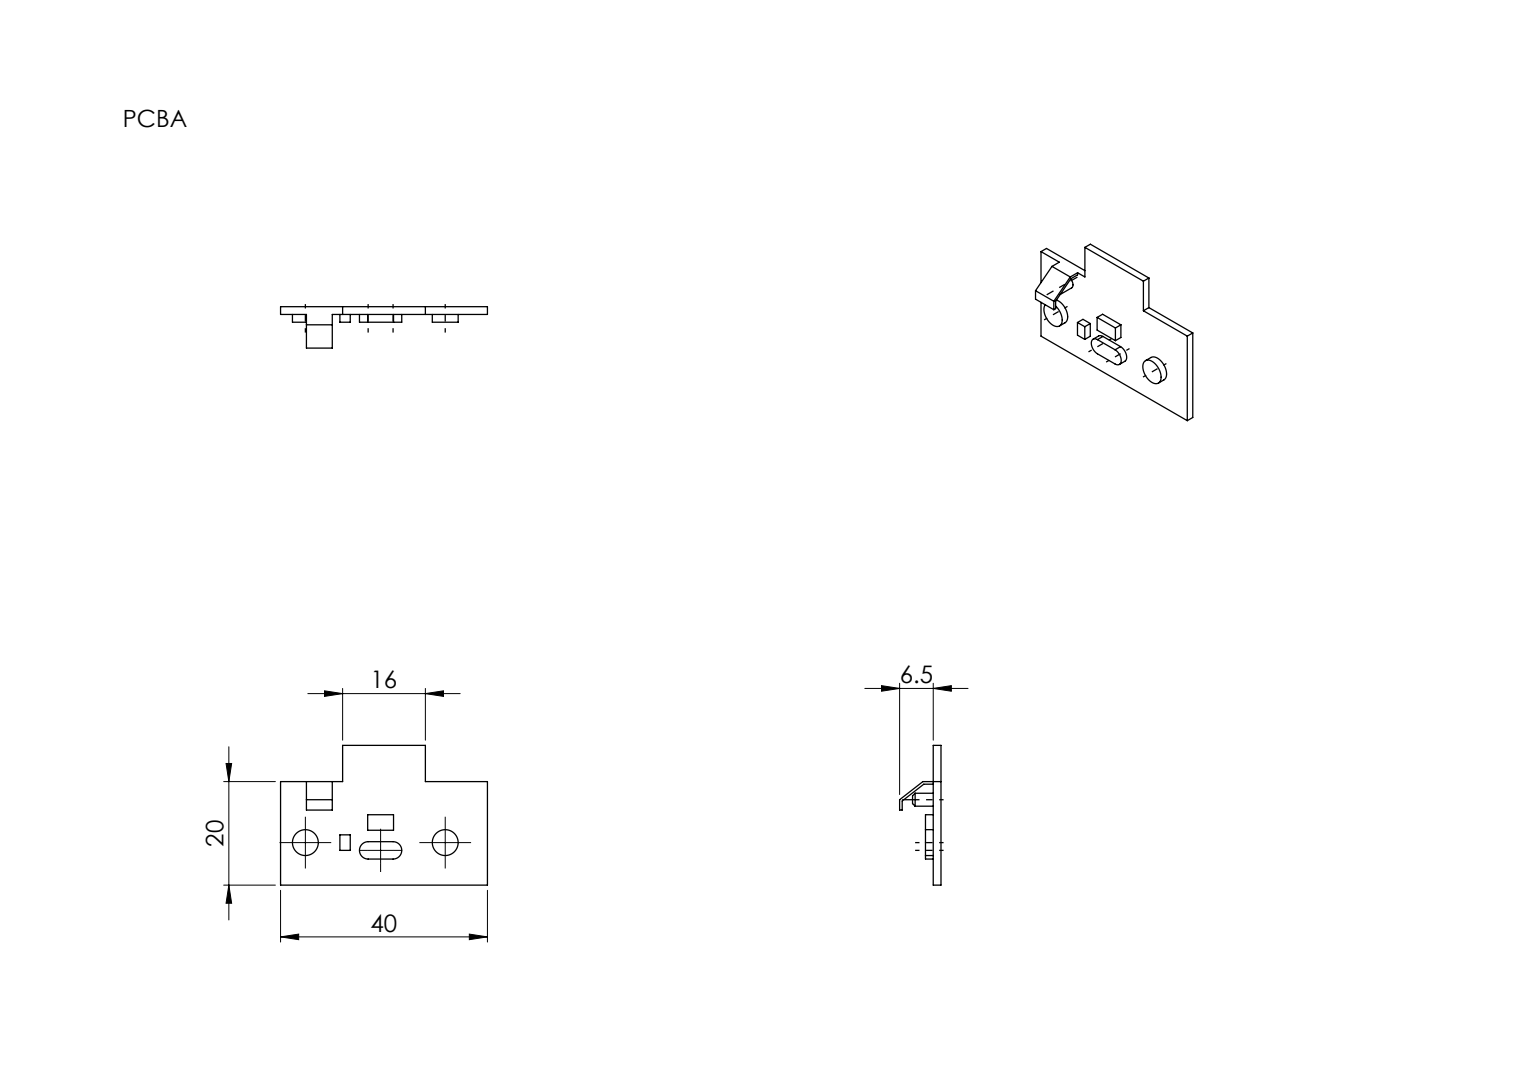
ISO-10303-21;
HEADER;
FILE_DESCRIPTION (('STEP AP214'),
    '1' );
FILE_NAME ('pcba.step',
    '2026-10-08T14:41:38',
    ( '' ),
    ( '' ),
    'SwSTEP 2.0',
    'SolidWorks 2026',
    '' );
FILE_SCHEMA (( 'AUTOMOTIVE_DESIGN' ));
ENDSEC;

DATA;
#13=DIRECTION ( 'NONE',  ( -1.000000000000000000, -2.168404344971008868E-16, 0.000000000000000000 ) ) ;
#56=ADVANCED_FACE ( 'NONE', ( #13399 ), #17297, .T. ) ;
#65=DIRECTION ( 'NONE',  ( 1.000000000000000000, 0.000000000000000000, 0.000000000000000000 ) ) ;
#70=LINE ( 'NONE', #3095, #14117 ) ;
#72=VERTEX_POINT ( 'NONE', #4700 ) ;
#100=EDGE_LOOP ( 'NONE', ( #14836, #13611, #8992, #9930 ) ) ;
#134=DIRECTION ( 'NONE',  ( 0.000000000000000000, -1.000000000000000000, 0.000000000000000000 ) ) ;
#136=AXIS2_PLACEMENT_3D ( 'NONE', #17568, #5609, #6979 ) ;
#169=ADVANCED_FACE ( 'NONE', ( #13798 ), #17134, .T. ) ;
#190=ADVANCED_FACE ( 'NONE', ( #565 ), #6556, .T. ) ;
#192=AXIS2_PLACEMENT_3D ( 'NONE', #9179, #627, #10638 ) ;
#199=DIRECTION ( 'NONE',  ( 0.000000000000000000, 1.000000000000000000, -0.000000000000000000 ) ) ;
#210=CIRCLE ( 'NONE', #18070, 1.678500596222258556 ) ;
#241=UNCERTAINTY_MEASURE_WITH_UNIT (LENGTH_MEASURE( 1.000000000000000082E-05 ), #5755, 'distance_accuracy_value', 'NONE');
#281=LINE ( 'NONE', #12431, #10985 ) ;
#287=EDGE_LOOP ( 'NONE', ( #9707, #2750, #19384, #14817 ) ) ;
#301=VERTEX_POINT ( 'NONE', #18229 ) ;
#308=CARTESIAN_POINT ( 'NONE',  ( -3.155775640247338920, -41.39960408384398249, 3.000000000000000000 ) ) ;
#326=VECTOR ( 'NONE', #8831, 1000.000000000000000 ) ;
#330=EDGE_LOOP ( 'NONE', ( #1279, #8353, #4314, #6562 ) ) ;
#363=EDGE_LOOP ( 'NONE', ( #16148, #12127, #5971, #7441 ) ) ;
#376=ORIENTED_EDGE ( 'NONE', *, *, #4655, .F. ) ;
#414=CARTESIAN_POINT ( 'NONE',  ( -15.20357423236093375, -43.78611686177728046, 3.000000000000000000 ) ) ;
#440=ORIENTED_EDGE ( 'NONE', *, *, #14376, .F. ) ;
#446=DIRECTION ( 'NONE',  ( -1.000000000000000000, 0.000000000000000000, -0.000000000000000000 ) ) ;
#452=LINE ( 'NONE', #1930, #15081 ) ;
#456=DIRECTION ( 'NONE',  ( -0.000000000000000000, -0.000000000000000000, -1.000000000000000000 ) ) ;
#471=DIRECTION ( 'NONE',  ( 0.000000000000000000, -1.000000000000000000, 0.000000000000000000 ) ) ;
#492=ORIENTED_EDGE ( 'NONE', *, *, #2758, .T. ) ;
#507=DIRECTION ( 'NONE',  ( 0.000000000000000000, -1.000000000000000000, 0.000000000000000000 ) ) ;
#508=CARTESIAN_POINT ( 'NONE',  ( 20.00000000000000355, -32.00000000000000711, 1.500000000000000000 ) ) ;
#519=CARTESIAN_POINT ( 'NONE',  ( -10.00000000000000000, -17.18313764714974923, -16.36466261444977377 ) ) ;
#558=DIRECTION ( 'NONE',  ( -1.000000000000000000, 0.000000000000000000, -0.000000000000000000 ) ) ;
#565=FACE_OUTER_BOUND ( 'NONE', #15076, .T. ) ;
#567=DIRECTION ( 'NONE',  ( 0.000000000000000000, 1.000000000000000000, 0.000000000000000000 ) ) ;
#573=ORIENTED_EDGE ( 'NONE', *, *, #9984, .T. ) ;
#578=VERTEX_POINT ( 'NONE', #19174 ) ;
#614=ORIENTED_EDGE ( 'NONE', *, *, #3279, .F. ) ;
#627=DIRECTION ( 'NONE',  ( 0.000000000000000000, 0.000000000000000000, 1.000000000000000000 ) ) ;
#747=CARTESIAN_POINT ( 'NONE',  ( 0.000000000000000000, 0.000000000000000000, 3.000000000000000000 ) ) ;
#752=CARTESIAN_POINT ( 'NONE',  ( -1.485306817036799787, -32.50000000000000711, -3.000000000000000000 ) ) ;
#754=DIRECTION ( 'NONE',  ( 1.000000000000000000, 0.000000000000000000, 0.000000000000000000 ) ) ;
#763=VERTEX_POINT ( 'NONE', #6340 ) ;
#793=VERTEX_POINT ( 'NONE', #18588 ) ;
#811=SURFACE_SIDE_STYLE ('',( #2189 ) ) ;
#826=LINE ( 'NONE', #14446, #4346 ) ;
#833=DIRECTION ( 'NONE',  ( -0.000000000000000000, -0.000000000000000000, -1.000000000000000000 ) ) ;
#850=CARTESIAN_POINT ( 'NONE',  ( -12.50000000000000000, -35.50000000000000000, 5.500000000000000000 ) ) ;
#856=VERTEX_POINT ( 'NONE', #12774 ) ;
#873=PLANE ( 'NONE',  #1854 ) ;
#874=PLANE ( 'NONE',  #924 ) ;
#878=CARTESIAN_POINT ( 'NONE',  ( -6.528048594804060301, -45.28611686177728046, 3.000000000000000000 ) ) ;
#893=EDGE_LOOP ( 'NONE', ( #6187, #11365, #9315, #5304 ) ) ;
#924=AXIS2_PLACEMENT_3D ( 'NONE', #9416, #11075, #6488 ) ;
#938=EDGE_LOOP ( 'NONE', ( #12819, #19041, #5593, #2064 ) ) ;
#947=VECTOR ( 'NONE', #14495, 1000.000000000000000 ) ;
#961=LINE ( 'NONE', #13293, #11013 ) ;
#974=FACE_OUTER_BOUND ( 'NONE', #10751, .T. ) ;
#988=EDGE_CURVE ( 'NONE', #18409, #8629, #826, .T. ) ;
#997=CARTESIAN_POINT ( 'NONE',  ( -6.528048594804062965, -42.28611686177728046, 3.000000000000000000 ) ) ;
#1008=DIRECTION ( 'NONE',  ( 0.000000000000000000, 0.000000000000000000, 1.000000000000000000 ) ) ;
#1021=DIRECTION ( 'NONE',  ( -1.000000000000000000, -0.000000000000000000, -0.000000000000000000 ) ) ;
#1027=DIRECTION ( 'NONE',  ( 0.000000000000000000, -0.000000000000000000, 1.000000000000000000 ) ) ;
#1060=ADVANCED_FACE ( 'NONE', ( #19255 ), #2675, .F. ) ;
#1110=EDGE_CURVE ( 'NONE', #18251, #11621, #16207, .T. ) ;
#1111=CARTESIAN_POINT ( 'NONE',  ( 1.844224359752661968, -41.39960408384398249, 3.000000000000000000 ) ) ;
#1239=CARTESIAN_POINT ( 'NONE',  ( -15.00000000000000000, -32.00000000000000711, 1.500000000000000000 ) ) ;
#1246=ORIENTED_EDGE ( 'NONE', *, *, #7374, .T. ) ;
#1269=DIRECTION ( 'NONE',  ( -0.000000000000000000, -0.000000000000000000, -1.000000000000000000 ) ) ;
#1279=ORIENTED_EDGE ( 'NONE', *, *, #12979, .F. ) ;
#1294=VECTOR ( 'NONE', #5042, 1000.000000000000000 ) ;
#1303=CARTESIAN_POINT ( 'NONE',  ( -15.00000000000000000, -32.50000000000000711, -3.000000000000000000 ) ) ;
#1311=DIRECTION ( 'NONE',  ( -1.000000000000000000, -0.000000000000000000, -0.000000000000000000 ) ) ;
#1316=CARTESIAN_POINT ( 'NONE',  ( 20.00000000000000355, -32.00000000000000711, 1.500000000000000000 ) ) ;
#1345=EDGE_LOOP ( 'NONE', ( #11317, #15399, #5466, #15948 ) ) ;
#1361=EDGE_CURVE ( 'NONE', #8629, #9506, #8151, .T. ) ;
#1366=ADVANCED_FACE ( 'NONE', ( #8332 ), #874, .F. ) ;
#1372=VERTEX_POINT ( 'NONE', #16983 ) ;
#1403=CARTESIAN_POINT ( 'NONE',  ( -1.485306817036799787, -32.50000000000001421, 3.328446124929187455 ) ) ;
#1407=ORIENTED_EDGE ( 'NONE', *, *, #2893, .F. ) ;
#1412=CARTESIAN_POINT ( 'NONE',  ( 0.000000000000000000, -32.00000000000000711, 1.500000000000000000 ) ) ;
#1413=ADVANCED_FACE ( 'NONE', ( #974 ), #5772, .F. ) ;
#1420=AXIS2_PLACEMENT_3D ( 'NONE', #8834, #4433, #7561 ) ;
#1430=AXIS2_PLACEMENT_3D ( 'NONE', #414, #15121, #12459 ) ;
#1446=DIRECTION ( 'NONE',  ( 0.000000000000000000, -1.000000000000000000, 0.000000000000000000 ) ) ;
#1482=LINE ( 'NONE', #6087, #16267 ) ;
#1488=ORIENTED_EDGE ( 'NONE', *, *, #13083, .F. ) ;
#1515=FACE_OUTER_BOUND ( 'NONE', #9786, .T. ) ;
#1530=DIRECTION ( 'NONE',  ( -0.000000000000000000, -0.000000000000000000, -1.000000000000000000 ) ) ;
#1538=CARTESIAN_POINT ( 'NONE',  ( -1.485306817036799787, -37.50000000000000000, 7.999999999999996447 ) ) ;
#1545=FACE_OUTER_BOUND ( 'NONE', #11575, .T. ) ;
#1569=EDGE_CURVE ( 'NONE', #18409, #6170, #16064, .T. ) ;
#1585=LINE ( 'NONE', #2849, #326 ) ;
#1612=FACE_OUTER_BOUND ( 'NONE', #16172, .T. ) ;
#1614=DIRECTION ( 'NONE',  ( 0.000000000000000000, -0.000000000000000000, -1.000000000000000000 ) ) ;
#1647=VERTEX_POINT ( 'NONE', #6265 ) ;
#1676=CYLINDRICAL_SURFACE ( 'NONE', #9076, 1.678500596222258556 ) ;
#1707=CYLINDRICAL_SURFACE ( 'NONE', #11087, 2.500000000000000444 ) ;
#1709=CARTESIAN_POINT ( 'NONE',  ( 8.000000000000003553, -25.00000000000000711, 0.000000000000000000 ) ) ;
#1764=ORIENTED_EDGE ( 'NONE', *, *, #10465, .T. ) ;
#1791=AXIS2_PLACEMENT_3D ( 'NONE', #13713, #4815, #7646 ) ;
#1792=DIRECTION ( 'NONE',  ( -0.000000000000000000, -1.000000000000000000, -0.000000000000000000 ) ) ;
#1802=CARTESIAN_POINT ( 'NONE',  ( -7.999999999999996447, 0.000000000000000000, 1.500000000000000000 ) ) ;
#1821=CARTESIAN_POINT ( 'NONE',  ( -10.00000000000000000, -32.00000000000000711, -3.000000000000000000 ) ) ;
#1826=CARTESIAN_POINT ( 'NONE',  ( 9.339266095310328808, -43.78611686177728046, 3.000000000000000000 ) ) ;
#1842=ORIENTED_EDGE ( 'NONE', *, *, #1110, .T. ) ;
#1846=EDGE_LOOP ( 'NONE', ( #6833, #19010 ) ) ;
#1849=CARTESIAN_POINT ( 'NONE',  ( -8.528048594804062077, -45.28611686177728046, 1.500000000000000000 ) ) ;
#1851=ADVANCED_FACE ( 'NONE', ( #15380 ), #1951, .T. ) ;
#1854=AXIS2_PLACEMENT_3D ( 'NONE', #6851, #17256, #7042 ) ;
#1864=ORIENTED_EDGE ( 'NONE', *, *, #15200, .T. ) ;
#1868=DIRECTION ( 'NONE',  ( -1.000000000000000000, 0.000000000000000000, 0.000000000000000000 ) ) ;
#1881=VECTOR ( 'NONE', #2671, 1000.000000000000000 ) ;
#1899=ORIENTED_EDGE ( 'NONE', *, *, #3507, .T. ) ;
#1900=VECTOR ( 'NONE', #1311, 1000.000000000000000 ) ;
#1930=CARTESIAN_POINT ( 'NONE',  ( -15.00000000000000000, 0.000000000000000000, 7.499999999999995559 ) ) ;
#1948=ORIENTED_EDGE ( 'NONE', *, *, #18362, .F. ) ;
#1951=PLANE ( 'NONE',  #9058 ) ;
#1972=ORIENTED_EDGE ( 'NONE', *, *, #16364, .F. ) ;
#1981=CARTESIAN_POINT ( 'NONE',  ( -6.528048594804062965, -42.28611686177728046, 1.500000000000000000 ) ) ;
#2003=EDGE_CURVE ( 'NONE', #6543, #16247, #14565, .T. ) ;
#2024=EDGE_LOOP ( 'NONE', ( #17054, #11269, #614, #1864 ) ) ;
#2052=VERTEX_POINT ( 'NONE', #10135 ) ;
#2064=ORIENTED_EDGE ( 'NONE', *, *, #8373, .F. ) ;
#2076=LINE ( 'NONE', #12065, #18989 ) ;
#2083=CARTESIAN_POINT ( 'NONE',  ( 0.000000000000000000, -32.00000000000000711, 1.500000000000000000 ) ) ;
#2100=AXIS2_PLACEMENT_3D ( 'NONE', #12458, #507, #9517 ) ;
#2118=DIRECTION ( 'NONE',  ( 8.673617379884027583E-16, -1.000000000000000000, 0.000000000000000000 ) ) ;
#2133=ORIENTED_EDGE ( 'NONE', *, *, #10715, .T. ) ;
#2157=EDGE_LOOP ( 'NONE', ( #18218, #13220, #5391, #13980, #3183 ) ) ;
#2169=CARTESIAN_POINT ( 'NONE',  ( -10.00000000000000000, -37.50000000000000000, -3.000000000000000000 ) ) ;
#2189=SURFACE_STYLE_FILL_AREA ( #8271 ) ;
#2190=DIRECTION ( 'NONE',  ( -1.000000000000000000, -0.000000000000000000, -0.000000000000000000 ) ) ;
#2193=ORIENTED_EDGE ( 'NONE', *, *, #10563, .F. ) ;
#2199=EDGE_CURVE ( 'NONE', #3007, #4393, #13379, .T. ) ;
#2229=DIRECTION ( 'NONE',  ( 0.000000000000000000, 0.6139406135149196864, -0.7893522173763268812 ) ) ;
#2259=DIRECTION ( 'NONE',  ( 0.000000000000000000, -1.000000000000000000, 0.000000000000000000 ) ) ;
#2267=PLANE ( 'NONE',  #2100 ) ;
#2268=CARTESIAN_POINT ( 'NONE',  ( -8.528048594804062077, -42.28611686177728046, 1.500000000000000000 ) ) ;
#2282=DIRECTION ( 'NONE',  ( 0.000000000000000000, 0.000000000000000000, 1.000000000000000000 ) ) ;
#2286=( NAMED_UNIT ( * ) PLANE_ANGLE_UNIT ( ) SI_UNIT ( $, .RADIAN. ) );
#2321=CARTESIAN_POINT ( 'NONE',  ( -6.528048594804062965, -42.28611686177728046, 3.000000000000000000 ) ) ;
#2326=ADVANCED_FACE ( 'NONE', ( #4674 ), #12498, .F. ) ;
#2332=ORIENTED_EDGE ( 'NONE', *, *, #3099, .F. ) ;
#2339=AXIS2_PLACEMENT_3D ( 'NONE', #16822, #8282, #446 ) ;
#2352=EDGE_CURVE ( 'NONE', #18051, #793, #7911, .T. ) ;
#2430=DIRECTION ( 'NONE',  ( -1.000000000000000000, 0.000000000000000000, -0.000000000000000000 ) ) ;
#2438=DIRECTION ( 'NONE',  ( 0.000000000000000000, -0.000000000000000000, 1.000000000000000000 ) ) ;
#2453=ADVANCED_FACE ( 'NONE', ( #4872 ), #12405, .F. ) ;
#2457=EDGE_LOOP ( 'NONE', ( #10247, #3332 ) ) ;
#2468=DIRECTION ( 'NONE',  ( 0.000000000000000000, 0.000000000000000000, 1.000000000000000000 ) ) ;
#2472=VECTOR ( 'NONE', #4112, 1000.000000000000000 ) ;
#2479=DIRECTION ( 'NONE',  ( -0.000000000000000000, 0.000000000000000000, 1.000000000000000000 ) ) ;
#2490=CARTESIAN_POINT ( 'NONE',  ( -7.999999999999996447, -25.00000000000000711, 0.000000000000000000 ) ) ;
#2505=VECTOR ( 'NONE', #6895, 1000.000000000000000 ) ;
#2511=AXIS2_PLACEMENT_3D ( 'NONE', #9422, #12649, #15416 ) ;
#2513=ORIENTED_EDGE ( 'NONE', *, *, #12979, .T. ) ;
#2535=LINE ( 'NONE', #8517, #17195 ) ;
#2539=VECTOR ( 'NONE', #4970, 1000.000000000000000 ) ;
#2542=ORIENTED_EDGE ( 'NONE', *, *, #17103, .F. ) ;
#2570=ORIENTED_EDGE ( 'NONE', *, *, #2199, .T. ) ;
#2580=DIRECTION ( 'NONE',  ( 0.000000000000000000, 0.000000000000000000, 1.000000000000000000 ) ) ;
#2589=CARTESIAN_POINT ( 'NONE',  ( -0.000000000000000000, -32.00000000000000711, 0.000000000000000000 ) ) ;
#2604=CARTESIAN_POINT ( 'NONE',  ( 5.421010862427523748E-15, -25.00000000000000711, 1.500000000000000000 ) ) ;
#2630=EDGE_LOOP ( 'NONE', ( #10961, #6937, #15456, #10655 ) ) ;
#2639=VECTOR ( 'NONE', #11984, 1000.000000000000000 ) ;
#2642=DIRECTION ( 'NONE',  ( -0.000000000000000000, -0.000000000000000000, -1.000000000000000000 ) ) ;
#2650=DIRECTION ( 'NONE',  ( 1.000000000000000000, 0.000000000000000000, 0.000000000000000000 ) ) ;
#2661=CARTESIAN_POINT ( 'NONE',  ( 11.83926609531033058, -43.78611686177728046, 1.500000000000000000 ) ) ;
#2665=VECTOR ( 'NONE', #8253, 1000.000000000000000 ) ;
#2671=DIRECTION ( 'NONE',  ( -0.000000000000000000, -1.000000000000000000, -0.000000000000000000 ) ) ;
#2675=PLANE ( 'NONE',  #9957 ) ;
#2689=DIRECTION ( 'NONE',  ( -1.000000000000000000, -0.000000000000000000, -0.000000000000000000 ) ) ;
#2710=ORIENTED_EDGE ( 'NONE', *, *, #11748, .T. ) ;
#2733=CARTESIAN_POINT ( 'NONE',  ( -4.744034285469996171, -45.28611686177728046, 1.500000000000000000 ) ) ;
#2734=LINE ( 'NONE', #878, #17090 ) ;
#2750=ORIENTED_EDGE ( 'NONE', *, *, #7416, .T. ) ;
#2756=CARTESIAN_POINT ( 'NONE',  ( 11.83926609531033058, -43.78611686177728046, 3.000000000000000000 ) ) ;
#2758=EDGE_CURVE ( 'NONE', #15605, #18409, #18146, .T. ) ;
#2759=DIRECTION ( 'NONE',  ( -1.000000000000000000, -0.000000000000000000, -0.000000000000000000 ) ) ;
#2809=VECTOR ( 'NONE', #18445, 1000.000000000000000 ) ;
#2829=CARTESIAN_POINT ( 'NONE',  ( -15.00000000000000000, -37.50000000000000000, 7.999999999999996447 ) ) ;
#2849=CARTESIAN_POINT ( 'NONE',  ( -13.75000000000000000, -35.50000000000000000, 5.500000000000000000 ) ) ;
#2853=DIRECTION ( 'NONE',  ( -0.000000000000000000, -0.000000000000000000, -1.000000000000000000 ) ) ;
#2859=DIRECTION ( 'NONE',  ( 0.000000000000000000, -0.000000000000000000, 1.000000000000000000 ) ) ;
#2885=ORIENTED_EDGE ( 'NONE', *, *, #11765, .F. ) ;
#2893=EDGE_CURVE ( 'NONE', #18722, #72, #1482, .T. ) ;
#2902=ADVANCED_FACE ( 'NONE', ( #10578 ), #1676, .T. ) ;
#2934=EDGE_CURVE ( 'NONE', #13522, #8266, #17844, .T. ) ;
#2958=DIRECTION ( 'NONE',  ( -0.000000000000000000, -0.000000000000000000, -1.000000000000000000 ) ) ;
#2966=DIRECTION ( 'NONE',  ( 0.000000000000000000, 1.000000000000000000, -0.000000000000000000 ) ) ;
#2992=DIRECTION ( 'NONE',  ( -0.000000000000000000, -0.000000000000000000, -1.000000000000000000 ) ) ;
#2997=CARTESIAN_POINT ( 'NONE',  ( -3.155775640247338920, -38.39960408384397539, 3.000000000000000000 ) ) ;
#3007=VERTEX_POINT ( 'NONE', #15398 ) ;
#3050=DIRECTION ( 'NONE',  ( -1.000000000000000000, 0.000000000000000000, 0.000000000000000000 ) ) ;
#3074=DIRECTION ( 'NONE',  ( -0.000000000000000000, -0.000000000000000000, -1.000000000000000000 ) ) ;
#3090=CARTESIAN_POINT ( 'NONE',  ( -17.70357423236093553, -43.78611686177728046, 3.000000000000000000 ) ) ;
#3095=CARTESIAN_POINT ( 'NONE',  ( -19.99999999999999645, -52.00000000000000711, 1.500000000000000000 ) ) ;
#3099=EDGE_CURVE ( 'NONE', #9583, #9953, #9783, .T. ) ;
#3100=VERTEX_POINT ( 'NONE', #9874 ) ;
#3104=SHAPE_REPRESENTATION_RELATIONSHIP ( 'NONE' , 'NONE' ,  #9996, #4072 ) ;
#3183=ORIENTED_EDGE ( 'NONE', *, *, #5411, .F. ) ;
#3193=DIRECTION ( 'NONE',  ( 0.000000000000000000, 1.000000000000000000, -0.000000000000000000 ) ) ;
#3204=DIRECTION ( 'NONE',  ( -1.000000000000000000, 0.000000000000000000, 0.000000000000000000 ) ) ;
#3236=VERTEX_POINT ( 'NONE', #13003 ) ;
#3257=DIRECTION ( 'NONE',  ( 1.000000000000000000, 0.000000000000000000, -0.000000000000000000 ) ) ;
#3273=EDGE_CURVE ( 'NONE', #15565, #12155, #10108, .T. ) ;
#3278=DIRECTION ( 'NONE',  ( 1.000000000000000000, 0.000000000000000000, 0.000000000000000000 ) ) ;
#3279=EDGE_CURVE ( 'NONE', #856, #3523, #9719, .T. ) ;
#3281=DIRECTION ( 'NONE',  ( 1.000000000000000000, 0.000000000000000000, -0.000000000000000000 ) ) ;
#3330=VECTOR ( 'NONE', #7296, 1000.000000000000000 ) ;
#3331=CARTESIAN_POINT ( 'NONE',  ( 1.753982408753060440, -43.60761626555502346, 3.000000000000000000 ) ) ;
#3332=ORIENTED_EDGE ( 'NONE', *, *, #9838, .T. ) ;
#3336=ORIENTED_EDGE ( 'NONE', *, *, #9928, .F. ) ;
#3345=VECTOR ( 'NONE', #13543, 1000.000000000000000 ) ;
#3349=DIRECTION ( 'NONE',  ( 1.000000000000000000, 0.000000000000000000, 0.000000000000000000 ) ) ;
#3353=LINE ( 'NONE', #308, #9389 ) ;
#3397=VERTEX_POINT ( 'NONE', #11978 ) ;
#3402=ORIENTED_EDGE ( 'NONE', *, *, #4719, .F. ) ;
#3412=DIRECTION ( 'NONE',  ( -0.000000000000000000, -0.000000000000000000, -1.000000000000000000 ) ) ;
#3434=AXIS2_PLACEMENT_3D ( 'NONE', #12694, #18698, #18885 ) ;
#3491=VECTOR ( 'NONE', #6146, 1000.000000000000000 ) ;
#3498=( GEOMETRIC_REPRESENTATION_CONTEXT ( 3 ) GLOBAL_UNCERTAINTY_ASSIGNED_CONTEXT ( ( #10814 ) ) GLOBAL_UNIT_ASSIGNED_CONTEXT ( ( #17192, #2286, #12761 ) ) REPRESENTATION_CONTEXT ( 'NONE', 'WORKASPACE' ) );
#3507=EDGE_CURVE ( 'NONE', #4220, #13466, #10405, .T. ) ;
#3523=VERTEX_POINT ( 'NONE', #14935 ) ;
#3538=LINE ( 'NONE', #9507, #17512 ) ;
#3541=FACE_BOUND ( 'NONE', #7383, .T. ) ;
#3554=ORIENTED_EDGE ( 'NONE', *, *, #16920, .T. ) ;
#3578=FACE_OUTER_BOUND ( 'NONE', #11546, .T. ) ;
#3584=DIRECTION ( 'NONE',  ( -1.000000000000000000, 0.000000000000000000, 0.000000000000000000 ) ) ;
#3599=ORIENTED_EDGE ( 'NONE', *, *, #13350, .T. ) ;
#3604=CIRCLE ( 'NONE', #14551, 1.249999999999999334 ) ;
#3610=ADVANCED_FACE ( 'NONE', ( #12375 ), #13850, .T. ) ;
#3634=FACE_BOUND ( 'NONE', #5753, .T. ) ;
#3641=CARTESIAN_POINT ( 'NONE',  ( -19.99999999999999645, -52.00000000000000711, 1.500000000000000000 ) ) ;
#3650=EDGE_CURVE ( 'NONE', #4220, #4614, #13944, .T. ) ;
#3660=DIRECTION ( 'NONE',  ( -1.000000000000000000, -0.000000000000000000, -0.000000000000000000 ) ) ;
#3726=AXIS2_PLACEMENT_3D ( 'NONE', #7114, #5943, #65 ) ;
#3731=FACE_OUTER_BOUND ( 'NONE', #13883, .T. ) ;
#3747=ORIENTED_EDGE ( 'NONE', *, *, #12665, .T. ) ;
#3784=LINE ( 'NONE', #11315, #5515 ) ;
#3833=ORIENTED_EDGE ( 'NONE', *, *, #8201, .F. ) ;
#3845=DIRECTION ( 'NONE',  ( -1.000000000000000000, 0.000000000000000000, 0.000000000000000000 ) ) ;
#3853=DIRECTION ( 'NONE',  ( 0.000000000000000000, 0.000000000000000000, -1.000000000000000000 ) ) ;
#3874=CARTESIAN_POINT ( 'NONE',  ( 1.844224359752661968, -38.39960408384397539, 1.500000000000000000 ) ) ;
#3883=LINE ( 'NONE', #18704, #19103 ) ;
#3898=ORIENTED_EDGE ( 'NONE', *, *, #2003, .F. ) ;
#3902=( GEOMETRIC_REPRESENTATION_CONTEXT ( 3 ) GLOBAL_UNCERTAINTY_ASSIGNED_CONTEXT ( ( #241 ) ) GLOBAL_UNIT_ASSIGNED_CONTEXT ( ( #5755, #7124, #5955 ) ) REPRESENTATION_CONTEXT ( 'NONE', 'WORKASPACE' ) );
#3919=VECTOR ( 'NONE', #2853, 1000.000000000000000 ) ;
#3935=DIRECTION ( 'NONE',  ( 1.000000000000000000, 0.000000000000000000, -0.000000000000000000 ) ) ;
#3959=LINE ( 'NONE', #1316, #16106 ) ;
#3960=AXIS2_PLACEMENT_3D ( 'NONE', #14333, #2468, #6799 ) ;
#3994=ORIENTED_EDGE ( 'NONE', *, *, #18190, .F. ) ;
#4012=CARTESIAN_POINT ( 'NONE',  ( -3.065533689247737392, -46.96461745799954457, 1.500000000000000000 ) ) ;
#4015=ORIENTED_EDGE ( 'NONE', *, *, #16920, .F. ) ;
#4072=ADVANCED_BREP_SHAPE_REPRESENTATION ( '', ( #10198, #1791 ), #3902 ) ;
#4081=ADVANCED_FACE ( 'NONE', ( #12914 ), #17339, .T. ) ;
#4086=AXIS2_PLACEMENT_3D ( 'NONE', #17442, #14400, #11644 ) ;
#4100=DIRECTION ( 'NONE',  ( 1.000000000000000000, 0.000000000000000000, 0.000000000000000000 ) ) ;
#4110=CARTESIAN_POINT ( 'NONE',  ( 1.844224359752661968, -41.39960408384398249, 3.000000000000000000 ) ) ;
#4112=DIRECTION ( 'NONE',  ( 0.000000000000000000, -1.000000000000000000, 0.000000000000000000 ) ) ;
#4113=AXIS2_PLACEMENT_3D ( 'NONE', #13995, #3412, #18522 ) ;
#4116=DIRECTION ( 'NONE',  ( -0.000000000000000000, -0.000000000000000000, -1.000000000000000000 ) ) ;
#4120=ORIENTED_EDGE ( 'NONE', *, *, #17901, .F. ) ;
#4125=VECTOR ( 'NONE', #2259, 1000.000000000000000 ) ;
#4186=DIRECTION ( 'NONE',  ( 1.000000000000000000, 2.168404344971008868E-16, 0.000000000000000000 ) ) ;
#4204=ORIENTED_EDGE ( 'NONE', *, *, #3650, .F. ) ;
#4213=ORIENTED_EDGE ( 'NONE', *, *, #17059, .T. ) ;
#4220=VERTEX_POINT ( 'NONE', #17433 ) ;
#4294=ORIENTED_EDGE ( 'NONE', *, *, #15404, .F. ) ;
#4314=ORIENTED_EDGE ( 'NONE', *, *, #13597, .T. ) ;
#4335=VECTOR ( 'NONE', #5747, 1000.000000000000000 ) ;
#4346=VECTOR ( 'NONE', #1021, 1000.000000000000000 ) ;
#4356=LINE ( 'NONE', #8561, #15968 ) ;
#4393=VERTEX_POINT ( 'NONE', #4991 ) ;
#4403=CARTESIAN_POINT ( 'NONE',  ( -12.50000000000000000, -35.50000000000000000, 5.500000000000000000 ) ) ;
#4411=CARTESIAN_POINT ( 'NONE',  ( 1.844224359752661968, -41.39960408384398249, 1.500000000000000000 ) ) ;
#4418=EDGE_LOOP ( 'NONE', ( #8684, #4015, #16173, #12411 ) ) ;
#4421=VECTOR ( 'NONE', #4186, 1000.000000000000000 ) ;
#4433=DIRECTION ( 'NONE',  ( -1.000000000000000000, 0.000000000000000000, 0.000000000000000000 ) ) ;
#4480=DIRECTION ( 'NONE',  ( -1.000000000000000000, 0.000000000000000000, 0.000000000000000000 ) ) ;
#4513=ORIENTED_EDGE ( 'NONE', *, *, #10449, .F. ) ;
#4516=DIRECTION ( 'NONE',  ( 1.000000000000000000, 0.000000000000000000, 0.000000000000000000 ) ) ;
#4523=ORIENTED_EDGE ( 'NONE', *, *, #3273, .F. ) ;
#4558=CARTESIAN_POINT ( 'NONE',  ( -12.70357423236093197, -43.78611686177728046, 1.500000000000000000 ) ) ;
#4561=CONICAL_SURFACE ( 'NONE', #11427, 0.7500000000000006661, 0.7853981633974511656 ) ;
#4573=VECTOR ( 'NONE', #17419, 1000.000000000000000 ) ;
#4589=VECTOR ( 'NONE', #16413, 1000.000000000000000 ) ;
#4590=CARTESIAN_POINT ( 'NONE',  ( 0.000000000000000000, -32.00000000000000711, 1.500000000000000000 ) ) ;
#4607=ADVANCED_FACE ( 'NONE', ( #12615 ), #9764, .F. ) ;
#4614=VERTEX_POINT ( 'NONE', #5365 ) ;
#4640=DIRECTION ( 'NONE',  ( -1.000000000000000000, 0.000000000000000000, 0.000000000000000000 ) ) ;
#4655=EDGE_CURVE ( 'NONE', #17673, #6113, #3883, .T. ) ;
#4674=FACE_OUTER_BOUND ( 'NONE', #1345, .T. ) ;
#4697=EDGE_CURVE ( 'NONE', #16767, #12626, #11519, .T. ) ;
#4700=CARTESIAN_POINT ( 'NONE',  ( 20.00000000000000355, -52.00000000000000711, 0.000000000000000000 ) ) ;
#4705=CIRCLE ( 'NONE', #3434, 1.678500596222258556 ) ;
#4719=EDGE_CURVE ( 'NONE', #10078, #5590, #9712, .T. ) ;
#4735=LINE ( 'NONE', #16689, #14597 ) ;
#4742=VECTOR ( 'NONE', #16338, 1000.000000000000000 ) ;
#4745=ORIENTED_EDGE ( 'NONE', *, *, #14636, .F. ) ;
#4760=VECTOR ( 'NONE', #14395, 1000.000000000000000 ) ;
#4761=DIRECTION ( 'NONE',  ( 0.000000000000000000, -0.000000000000000000, -1.000000000000000000 ) ) ;
#4767=CARTESIAN_POINT ( 'NONE',  ( -12.50000000000000000, -35.50000000000000000, 5.500000000000000000 ) ) ;
#4771=VECTOR ( 'NONE', #11631, 1000.000000000000000 ) ;
#4785=CARTESIAN_POINT ( 'NONE',  ( -19.99999999999999645, 0.000000000000000000, 1.500000000000000000 ) ) ;
#4797=LINE ( 'NONE', #10746, #9252 ) ;
#4815=DIRECTION ( 'NONE',  ( 0.000000000000000000, 0.000000000000000000, 1.000000000000000000 ) ) ;
#4853=EDGE_CURVE ( 'NONE', #14478, #3100, #4356, .T. ) ;
#4869=LINE ( 'NONE', #8805, #11952 ) ;
#4872=FACE_OUTER_BOUND ( 'NONE', #11358, .T. ) ;
#4881=( NAMED_UNIT ( * ) PLANE_ANGLE_UNIT ( ) SI_UNIT ( $, .RADIAN. ) );
#4885=DIRECTION ( 'NONE',  ( 0.000000000000000000, 0.000000000000000000, -1.000000000000000000 ) ) ;
#4906=ORIENTED_EDGE ( 'NONE', *, *, #9838, .F. ) ;
#4926=CARTESIAN_POINT ( 'NONE',  ( -15.00000000000000000, 0.000000000000000000, 7.999999999999996447 ) ) ;
#4938=ORIENTED_EDGE ( 'NONE', *, *, #9001, .T. ) ;
#4942=CARTESIAN_POINT ( 'NONE',  ( -3.065533689247737392, -45.28611686177728046, 3.000000000000000000 ) ) ;
#4957=EDGE_LOOP ( 'NONE', ( #16348, #15769, #18237, #5779 ) ) ;
#4960=EDGE_CURVE ( 'NONE', #9953, #11135, #3353, .T. ) ;
#4970=DIRECTION ( 'NONE',  ( -1.000000000000000000, -0.000000000000000000, -0.000000000000000000 ) ) ;
#4991=CARTESIAN_POINT ( 'NONE',  ( -10.00000000000000000, -32.50000000000000711, 1.500000000000000444 ) ) ;
#5042=DIRECTION ( 'NONE',  ( 1.000000000000000000, 0.000000000000000000, 0.000000000000000000 ) ) ;
#5045=LINE ( 'NONE', #16712, #9211 ) ;
#5075=ORIENTED_EDGE ( 'NONE', *, *, #14964, .F. ) ;
#5095=ADVANCED_FACE ( 'NONE', ( #3541, #3634, #9510, #8059, #14020, #18915, #11253 ), #873, .T. ) ;
#5111=DIRECTION ( 'NONE',  ( 0.000000000000000000, 0.000000000000000000, 1.000000000000000000 ) ) ;
#5117=ORIENTED_EDGE ( 'NONE', *, *, #9278, .F. ) ;
#5139=EDGE_CURVE ( 'NONE', #10078, #16767, #2535, .T. ) ;
#5140=CYLINDRICAL_SURFACE ( 'NONE', #17219, 1.678500596222258556 ) ;
#5150=AXIS2_PLACEMENT_3D ( 'NONE', #2756, #7169, #4640 ) ;
#5159=LINE ( 'NONE', #17565, #12575 ) ;
#5165=VERTEX_POINT ( 'NONE', #11352 ) ;
#5172=ORIENTED_EDGE ( 'NONE', *, *, #18744, .T. ) ;
#5238=VECTOR ( 'NONE', #9926, 1000.000000000000000 ) ;
#5239=CARTESIAN_POINT ( 'NONE',  ( -7.999999999999996447, -25.00000000000000711, 1.500000000000000000 ) ) ;
#5272=LINE ( 'NONE', #9770, #4573 ) ;
#5273=VERTEX_POINT ( 'NONE', #12735 ) ;
#5283=CARTESIAN_POINT ( 'NONE',  ( -8.528048594804062077, -42.28611686177728046, 1.500000000000000000 ) ) ;
#5288=EDGE_CURVE ( 'NONE', #13466, #13503, #7334, .T. ) ;
#5293=LINE ( 'NONE', #4110, #4760 ) ;
#5303=LINE ( 'NONE', #2169, #6123 ) ;
#5304=ORIENTED_EDGE ( 'NONE', *, *, #12384, .F. ) ;
#5322=AXIS2_PLACEMENT_3D ( 'NONE', #6283, #5111, #7951 ) ;
#5329=LINE ( 'NONE', #11193, #15843 ) ;
#5332=EDGE_LOOP ( 'NONE', ( #376, #6836, #13310, #18830 ) ) ;
#5362=AXIS2_PLACEMENT_3D ( 'NONE', #8243, #17158, #2430 ) ;
#5365=CARTESIAN_POINT ( 'NONE',  ( -10.00000000000000000, -35.74454190283286437, 7.499999999999996447 ) ) ;
#5391=ORIENTED_EDGE ( 'NONE', *, *, #12620, .F. ) ;
#5410=ORIENTED_EDGE ( 'NONE', *, *, #5920, .F. ) ;
#5411=EDGE_CURVE ( 'NONE', #9204, #9159, #16575, .T. ) ;
#5415=DIRECTION ( 'NONE',  ( 0.000000000000000000, 0.000000000000000000, 1.000000000000000000 ) ) ;
#5423=SURFACE_STYLE_USAGE ( .BOTH. , #811 ) ;
#5424=DIRECTION ( 'NONE',  ( -1.000000000000000000, 0.000000000000000000, -0.000000000000000000 ) ) ;
#5466=ORIENTED_EDGE ( 'NONE', *, *, #4960, .F. ) ;
#5485=CARTESIAN_POINT ( 'NONE',  ( 0.000000000000000000, -52.00000000000000711, 1.500000000000000000 ) ) ;
#5502=PLANE ( 'NONE',  #11873 ) ;
#5504=PLANE ( 'NONE',  #14703 ) ;
#5515=VECTOR ( 'NONE', #833, 1000.000000000000000 ) ;
#5536=EDGE_CURVE ( 'NONE', #18722, #16082, #10240, .T. ) ;
#5537=LINE ( 'NONE', #13063, #5238 ) ;
#5549=EDGE_CURVE ( 'NONE', #15869, #5273, #10281, .T. ) ;
#5550=DIRECTION ( 'NONE',  ( 0.000000000000000000, 0.000000000000000000, 1.000000000000000000 ) ) ;
#5571=ORIENTED_EDGE ( 'NONE', *, *, #18746, .T. ) ;
#5590=VERTEX_POINT ( 'NONE', #3090 ) ;
#5593=ORIENTED_EDGE ( 'NONE', *, *, #18394, .T. ) ;
#5602=VECTOR ( 'NONE', #134, 1000.000000000000000 ) ;
#5609=DIRECTION ( 'NONE',  ( 0.000000000000000000, -0.7893522173763268812, -0.6139406135149196864 ) ) ;
#5620=CARTESIAN_POINT ( 'NONE',  ( 1.753982408753060440, -45.28611686177728046, 3.000000000000000000 ) ) ;
#5631=VECTOR ( 'NONE', #3193, 1000.000000000000000 ) ;
#5632=PLANE ( 'NONE',  #17125 ) ;
#5654=EDGE_CURVE ( 'NONE', #9953, #2052, #8874, .T. ) ;
#5666=VECTOR ( 'NONE', #17188, 1000.000000000000000 ) ;
#5679=CARTESIAN_POINT ( 'NONE',  ( -10.00000000000000000, 0.000000000000000000, 7.999999999999996447 ) ) ;
#5698=APPLICATION_CONTEXT ( 'automotive_design' ) ;
#5747=DIRECTION ( 'NONE',  ( -0.000000000000000000, -0.000000000000000000, -1.000000000000000000 ) ) ;
#5750=FACE_OUTER_BOUND ( 'NONE', #18016, .T. ) ;
#5753=EDGE_LOOP ( 'NONE', ( #7052, #16177 ) ) ;
#5755=( LENGTH_UNIT ( ) NAMED_UNIT ( * ) SI_UNIT ( .MILLI., .METRE. ) );
#5757=EDGE_LOOP ( 'NONE', ( #8418, #15963, #18726, #7772, #15025 ) ) ;
#5772=PLANE ( 'NONE',  #6256 ) ;
#5779=ORIENTED_EDGE ( 'NONE', *, *, #7396, .T. ) ;
#5790=LINE ( 'NONE', #8916, #13123 ) ;
#5798=CARTESIAN_POINT ( 'NONE',  ( 5.421010862427523748E-15, -25.00000000000000711, 1.500000000000000000 ) ) ;
#5834=ORIENTED_EDGE ( 'NONE', *, *, #5139, .F. ) ;
#5850=LINE ( 'NONE', #18008, #14427 ) ;
#5897=DIRECTION ( 'NONE',  ( -0.000000000000000000, -0.000000000000000000, -1.000000000000000000 ) ) ;
#5901=VECTOR ( 'NONE', #14960, 1000.000000000000000 ) ;
#5905=LINE ( 'NONE', #13438, #11771 ) ;
#5914=CARTESIAN_POINT ( 'NONE',  ( 20.00000000000000355, 0.000000000000000000, 0.000000000000000000 ) ) ;
#5916=CARTESIAN_POINT ( 'NONE',  ( -10.00000000000000000, -37.50000000000000000, 7.999999999999996447 ) ) ;
#5920=EDGE_CURVE ( 'NONE', #9490, #12155, #11957, .T. ) ;
#5925=FACE_OUTER_BOUND ( 'NONE', #9365, .T. ) ;
#5943=DIRECTION ( 'NONE',  ( 0.000000000000000000, 0.000000000000000000, 1.000000000000000000 ) ) ;
#5948=DIRECTION ( 'NONE',  ( 0.000000000000000000, 0.000000000000000000, 1.000000000000000000 ) ) ;
#5952=ORIENTED_EDGE ( 'NONE', *, *, #12623, .F. ) ;
#5954=CIRCLE ( 'NONE', #7191, 1.678500596222258556 ) ;
#5955=( NAMED_UNIT ( * ) SI_UNIT ( $, .STERADIAN. ) SOLID_ANGLE_UNIT ( ) );
#5966=EDGE_CURVE ( 'NONE', #15107, #15565, #5790, .T. ) ;
#5971=ORIENTED_EDGE ( 'NONE', *, *, #15317, .F. ) ;
#5983=CARTESIAN_POINT ( 'NONE',  ( 11.83926609531033058, -43.78611686177728046, 3.000000000000000000 ) ) ;
#5993=ORIENTED_EDGE ( 'NONE', *, *, #2893, .T. ) ;
#6008=DIRECTION ( 'NONE',  ( 1.000000000000000000, 0.000000000000000000, 0.000000000000000000 ) ) ;
#6025=DIRECTION ( 'NONE',  ( 0.000000000000000000, -1.000000000000000000, 0.000000000000000000 ) ) ;
#6053=EDGE_LOOP ( 'NONE', ( #15714, #14119, #18993, #14136 ) ) ;
#6058=ORIENTED_EDGE ( 'NONE', *, *, #17781, .T. ) ;
#6070=DIRECTION ( 'NONE',  ( 0.000000000000000000, 0.000000000000000000, 1.000000000000000000 ) ) ;
#6087=CARTESIAN_POINT ( 'NONE',  ( 20.00000000000000355, -52.00000000000000711, 1.500000000000000000 ) ) ;
#6096=FACE_OUTER_BOUND ( 'NONE', #11184, .T. ) ;
#6105=LINE ( 'NONE', #9033, #7721 ) ;
#6113=VERTEX_POINT ( 'NONE', #3874 ) ;
#6123=VECTOR ( 'NONE', #8158, 1000.000000000000000 ) ;
#6133=EDGE_CURVE ( 'NONE', #578, #9541, #4705, .T. ) ;
#6146=DIRECTION ( 'NONE',  ( -1.000000000000000000, 0.000000000000000000, 0.000000000000000000 ) ) ;
#6170=VERTEX_POINT ( 'NONE', #5916 ) ;
#6187=ORIENTED_EDGE ( 'NONE', *, *, #14376, .T. ) ;
#6199=EDGE_CURVE ( 'NONE', #19316, #16247, #11784, .T. ) ;
#6218=CARTESIAN_POINT ( 'NONE',  ( -7.999999999999996447, -32.00000000000000711, 1.500000000000000000 ) ) ;
#6249=VECTOR ( 'NONE', #7384, 1000.000000000000000 ) ;
#6256=AXIS2_PLACEMENT_3D ( 'NONE', #14593, #8807, #2438 ) ;
#6265=CARTESIAN_POINT ( 'NONE',  ( 14.33926609531033058, -43.78611686177728046, 1.500000000000000000 ) ) ;
#6276=ORIENTED_EDGE ( 'NONE', *, *, #17526, .F. ) ;
#6283=CARTESIAN_POINT ( 'NONE',  ( -12.50000000000000000, -35.50000000000000000, 5.500000000000000000 ) ) ;
#6326=CIRCLE ( 'NONE', #7897, 1.249999999999999334 ) ;
#6340=CARTESIAN_POINT ( 'NONE',  ( -11.25000000000000178, -35.50000000000000000, 5.000000000000003553 ) ) ;
#6345=DIRECTION ( 'NONE',  ( 0.000000000000000000, -1.000000000000000000, 0.000000000000000000 ) ) ;
#6365=DIRECTION ( 'NONE',  ( 0.000000000000000000, -0.000000000000000000, -1.000000000000000000 ) ) ;
#6366=ORIENTED_EDGE ( 'NONE', *, *, #3650, .T. ) ;
#6374=VERTEX_POINT ( 'NONE', #18379 ) ;
#6390=DIRECTION ( 'NONE',  ( 0.7071067811865495711, 8.659560562354957510E-17, -0.7071067811865455743 ) ) ;
#6401=VERTEX_POINT ( 'NONE', #6218 ) ;
#6415=CARTESIAN_POINT ( 'NONE',  ( 1.844224359752661968, -38.39960408384397539, 3.000000000000000000 ) ) ;
#6431=PLANE ( 'NONE',  #2339 ) ;
#6438=LINE ( 'NONE', #12406, #2539 ) ;
#6446=( LENGTH_UNIT ( ) NAMED_UNIT ( * ) SI_UNIT ( .MILLI., .METRE. ) );
#6464=CIRCLE ( 'NONE', #15842, 1.678500596222258556 ) ;
#6488=DIRECTION ( 'NONE',  ( 0.000000000000000000, -0.000000000000000000, -1.000000000000000000 ) ) ;
#6543=VERTEX_POINT ( 'NONE', #997 ) ;
#6544=ADVANCED_FACE ( 'NONE', ( #6973 ), #5140, .T. ) ;
#6546=EDGE_CURVE ( 'NONE', #10710, #9506, #9627, .T. ) ;
#6556=PLANE ( 'NONE',  #7242 ) ;
#6561=VECTOR ( 'NONE', #2992, 1000.000000000000000 ) ;
#6562=ORIENTED_EDGE ( 'NONE', *, *, #17065, .T. ) ;
#6577=ORIENTED_EDGE ( 'NONE', *, *, #6199, .T. ) ;
#6594=FACE_OUTER_BOUND ( 'NONE', #1846, .T. ) ;
#6598=ADVANCED_FACE ( 'NONE', ( #18849 ), #5504, .T. ) ;
#6619=VECTOR ( 'NONE', #3660, 1000.000000000000000 ) ;
#6625=CARTESIAN_POINT ( 'NONE',  ( -19.99999999999999645, -32.00000000000000711, 1.500000000000000000 ) ) ;
#6649=ORIENTED_EDGE ( 'NONE', *, *, #3507, .F. ) ;
#6651=CARTESIAN_POINT ( 'NONE',  ( -15.20357423236093375, -43.78611686177728046, 3.000000000000000000 ) ) ;
#6676=ORIENTED_EDGE ( 'NONE', *, *, #18362, .T. ) ;
#6701=PLANE ( 'NONE',  #136 ) ;
#6723=VECTOR ( 'NONE', #17999, 1000.000000000000000 ) ;
#6749=AXIS2_PLACEMENT_3D ( 'NONE', #747, #4885, #558 ) ;
#6772=EDGE_CURVE ( 'NONE', #5165, #17673, #19033, .T. ) ;
#6790=FACE_OUTER_BOUND ( 'NONE', #7339, .T. ) ;
#6799=DIRECTION ( 'NONE',  ( 1.000000000000000000, 0.000000000000000000, 0.000000000000000000 ) ) ;
#6830=DIRECTION ( 'NONE',  ( 0.000000000000000000, 0.000000000000000000, 1.000000000000000000 ) ) ;
#6833=ORIENTED_EDGE ( 'NONE', *, *, #10449, .T. ) ;
#6836=ORIENTED_EDGE ( 'NONE', *, *, #6772, .F. ) ;
#6851=CARTESIAN_POINT ( 'NONE',  ( 0.000000000000000000, 0.000000000000000000, 1.500000000000000000 ) ) ;
#6855=LINE ( 'NONE', #17733, #947 ) ;
#6870=ORIENTED_EDGE ( 'NONE', *, *, #17901, .T. ) ;
#6874=ORIENTED_EDGE ( 'NONE', *, *, #15356, .T. ) ;
#6877=CARTESIAN_POINT ( 'NONE',  ( -15.00000000000000000, -37.50000000000000000, -3.000000000000000000 ) ) ;
#6895=DIRECTION ( 'NONE',  ( 0.000000000000000000, -1.000000000000000000, 0.000000000000000000 ) ) ;
#6912=AXIS2_PLACEMENT_3D ( 'NONE', #11712, #3204, #5948 ) ;
#6937=ORIENTED_EDGE ( 'NONE', *, *, #17065, .F. ) ;
#6949=LINE ( 'NONE', #11351, #4125 ) ;
#6955=CYLINDRICAL_SURFACE ( 'NONE', #7375, 1.249999999999999334 ) ;
#6973=FACE_OUTER_BOUND ( 'NONE', #18226, .T. ) ;
#6979=DIRECTION ( 'NONE',  ( 0.000000000000000000, 0.6139406135149196864, -0.7893522173763268812 ) ) ;
#6980=FILL_AREA_STYLE_COLOUR ( '', #18541 ) ;
#6998=ADVANCED_FACE ( 'NONE', ( #1545 ), #18014, .F. ) ;
#7021=DIRECTION ( 'NONE',  ( 0.000000000000000000, 0.000000000000000000, 1.000000000000000000 ) ) ;
#7022=ORIENTED_EDGE ( 'NONE', *, *, #11228, .T. ) ;
#7041=DIRECTION ( 'NONE',  ( 0.000000000000000000, 0.000000000000000000, 1.000000000000000000 ) ) ;
#7042=DIRECTION ( 'NONE',  ( 1.000000000000000000, 0.000000000000000000, 0.000000000000000000 ) ) ;
#7048=AXIS2_PLACEMENT_3D ( 'NONE', #5798, #13428, #13 ) ;
#7052=ORIENTED_EDGE ( 'NONE', *, *, #9001, .F. ) ;
#7114=CARTESIAN_POINT ( 'NONE',  ( -12.50000000000000000, -35.50000000000000000, 1.500000000000000000 ) ) ;
#7117=DIRECTION ( 'NONE',  ( 1.000000000000000000, 0.000000000000000000, 0.000000000000000000 ) ) ;
#7118=DIRECTION ( 'NONE',  ( 1.000000000000000000, 0.000000000000000000, 0.000000000000000000 ) ) ;
#7124=( NAMED_UNIT ( * ) PLANE_ANGLE_UNIT ( ) SI_UNIT ( $, .RADIAN. ) );
#7136=CARTESIAN_POINT ( 'NONE',  ( -7.999999999999996447, 0.000000000000000000, 0.000000000000000000 ) ) ;
#7138=CARTESIAN_POINT ( 'NONE',  ( -15.00000000000000000, -32.00000000000000711, -3.000000000000000000 ) ) ;
#7142=DIRECTION ( 'NONE',  ( 0.000000000000000000, -0.000000000000000000, -1.000000000000000000 ) ) ;
#7169=DIRECTION ( 'NONE',  ( -0.000000000000000000, -0.000000000000000000, -1.000000000000000000 ) ) ;
#7184=CARTESIAN_POINT ( 'NONE',  ( 1.753982408753060440, -43.60761626555502346, 1.500000000000000000 ) ) ;
#7191=AXIS2_PLACEMENT_3D ( 'NONE', #12448, #14017, #3349 ) ;
#7242=AXIS2_PLACEMENT_3D ( 'NONE', #752, #471, #6365 ) ;
#7249=CARTESIAN_POINT ( 'NONE',  ( -12.50000000000000000, -35.50000000000000000, 5.500000000000000000 ) ) ;
#7266=ADVANCED_FACE ( 'NONE', ( #1515 ), #14841, .F. ) ;
#7288=DIRECTION ( 'NONE',  ( -1.000000000000000000, 0.000000000000000000, 0.000000000000000000 ) ) ;
#7296=DIRECTION ( 'NONE',  ( -0.000000000000000000, -1.000000000000000000, -0.000000000000000000 ) ) ;
#7334=LINE ( 'NONE', #7636, #16236 ) ;
#7339=EDGE_LOOP ( 'NONE', ( #8908, #9480 ) ) ;
#7368=PLANE ( 'NONE',  #18950 ) ;
#7374=EDGE_CURVE ( 'NONE', #13384, #3397, #18474, .T. ) ;
#7375=AXIS2_PLACEMENT_3D ( 'NONE', #12926, #18920, #11451 ) ;
#7383=EDGE_LOOP ( 'NONE', ( #17815, #2542 ) ) ;
#7384=DIRECTION ( 'NONE',  ( -8.673617379884027583E-16, 1.000000000000000000, 0.000000000000000000 ) ) ;
#7395=CARTESIAN_POINT ( 'NONE',  ( -8.528048594804062077, -42.28611686177728046, 3.000000000000000000 ) ) ;
#7396=EDGE_CURVE ( 'NONE', #11135, #3236, #16901, .T. ) ;
#7416=EDGE_CURVE ( 'NONE', #15605, #301, #14149, .T. ) ;
#7428=ORIENTED_EDGE ( 'NONE', *, *, #11864, .F. ) ;
#7441=ORIENTED_EDGE ( 'NONE', *, *, #2003, .T. ) ;
#7444=CARTESIAN_POINT ( 'NONE',  ( -6.528048594804060301, -45.28611686177728046, 1.500000000000000000 ) ) ;
#7458=PLANE ( 'NONE',  #1420 ) ;
#7466=EDGE_CURVE ( 'NONE', #9583, #6113, #11189, .T. ) ;
#7477=ORIENTED_EDGE ( 'NONE', *, *, #11864, .T. ) ;
#7532=AXIS2_PLACEMENT_3D ( 'NONE', #4590, #1446, #19383 ) ;
#7561=DIRECTION ( 'NONE',  ( 0.000000000000000000, 0.000000000000000000, 1.000000000000000000 ) ) ;
#7570=FACE_OUTER_BOUND ( 'NONE', #11923, .T. ) ;
#7573=LINE ( 'NONE', #1303, #3345 ) ;
#7582=ORIENTED_EDGE ( 'NONE', *, *, #17526, .T. ) ;
#7636=CARTESIAN_POINT ( 'NONE',  ( -15.00000000000000000, -17.18313764714974923, -16.36466261444977377 ) ) ;
#7646=DIRECTION ( 'NONE',  ( 1.000000000000000000, 0.000000000000000000, 0.000000000000000000 ) ) ;
#7647=ORIENTED_EDGE ( 'NONE', *, *, #18637, .F. ) ;
#7657=ORIENTED_EDGE ( 'NONE', *, *, #18637, .T. ) ;
#7713=CARTESIAN_POINT ( 'NONE',  ( 1.844224359752661968, -41.39960408384398249, 3.000000000000000000 ) ) ;
#7721=VECTOR ( 'NONE', #2958, 1000.000000000000000 ) ;
#7760=CARTESIAN_POINT ( 'NONE',  ( -3.065533689247737392, -45.28611686177728046, 3.000000000000000000 ) ) ;
#7772=ORIENTED_EDGE ( 'NONE', *, *, #3279, .T. ) ;
#7781=CARTESIAN_POINT ( 'NONE',  ( 8.000000000000003553, -32.00000000000000711, 0.000000000000000000 ) ) ;
#7818=PRESENTATION_STYLE_ASSIGNMENT (( #18411 ) ) ;
#7848=ORIENTED_EDGE ( 'NONE', *, *, #4655, .T. ) ;
#7884=EDGE_LOOP ( 'NONE', ( #573, #14627, #2513, #17197, #14828, #13816, #7428, #3747 ) ) ;
#7897=AXIS2_PLACEMENT_3D ( 'NONE', #15256, #12106, #14072 ) ;
#7911=LINE ( 'NONE', #1826, #8711 ) ;
#7918=ORIENTED_EDGE ( 'NONE', *, *, #8373, .T. ) ;
#7936=CARTESIAN_POINT ( 'NONE',  ( -10.00000000000000000, 0.000000000000000000, -3.000000000000000000 ) ) ;
#7951=DIRECTION ( 'NONE',  ( 1.000000000000000000, 0.000000000000000000, 0.000000000000000000 ) ) ;
#7956=DIRECTION ( 'NONE',  ( -0.000000000000000000, -0.000000000000000000, -1.000000000000000000 ) ) ;
#7973=VERTEX_POINT ( 'NONE', #1849 ) ;
#7988=EDGE_CURVE ( 'NONE', #9541, #856, #281, .T. ) ;
#8006=DIRECTION ( 'NONE',  ( -0.000000000000000000, -0.000000000000000000, -1.000000000000000000 ) ) ;
#8017=SURFACE_STYLE_FILL_AREA ( #10742 ) ;
#8019=EDGE_LOOP ( 'NONE', ( #4906, #11626, #440, #18176 ) ) ;
#8045=VERTEX_POINT ( 'NONE', #12236 ) ;
#8059=FACE_BOUND ( 'NONE', #4418, .T. ) ;
#8072=DIRECTION ( 'NONE',  ( -1.000000000000000000, 0.000000000000000000, 0.000000000000000000 ) ) ;
#8094=CARTESIAN_POINT ( 'NONE',  ( -15.00000000000000000, -32.50000000000000711, 1.500000000000000000 ) ) ;
#8126=CARTESIAN_POINT ( 'NONE',  ( 1.844224359752661968, -38.39960408384397539, 3.000000000000000000 ) ) ;
#8148=ORIENTED_EDGE ( 'NONE', *, *, #5536, .T. ) ;
#8151=LINE ( 'NONE', #4926, #16585 ) ;
#8158=DIRECTION ( 'NONE',  ( -0.000000000000000000, 0.000000000000000000, 1.000000000000000000 ) ) ;
#8161=LINE ( 'NONE', #2083, #12711 ) ;
#8170=AXIS2_PLACEMENT_3D ( 'NONE', #4942, #10899, #12284 ) ;
#8201=EDGE_CURVE ( 'NONE', #6401, #3007, #10537, .T. ) ;
#8235=ORIENTED_EDGE ( 'NONE', *, *, #13597, .F. ) ;
#8240=CARTESIAN_POINT ( 'NONE',  ( 1.753982408753060440, -45.28611686177728046, 3.000000000000000000 ) ) ;
#8243=CARTESIAN_POINT ( 'NONE',  ( -1.485306817036799787, 0.000000000000000000, 7.499999999999995559 ) ) ;
#8253=DIRECTION ( 'NONE',  ( -1.000000000000000000, -0.000000000000000000, -0.000000000000000000 ) ) ;
#8264=ORIENTED_EDGE ( 'NONE', *, *, #5536, .F. ) ;
#8266=VERTEX_POINT ( 'NONE', #10136 ) ;
#8271=FILL_AREA_STYLE ('',( #6980 ) ) ;
#8273=FACE_OUTER_BOUND ( 'NONE', #16070, .T. ) ;
#8282=DIRECTION ( 'NONE',  ( 0.000000000000000000, 0.000000000000000000, -1.000000000000000000 ) ) ;
#8301=CARTESIAN_POINT ( 'NONE',  ( -15.20357423236093375, -43.78611686177728046, 1.500000000000000000 ) ) ;
#8332=FACE_OUTER_BOUND ( 'NONE', #363, .T. ) ;
#8341=EDGE_LOOP ( 'NONE', ( #14213, #1407, #8148, #17870 ) ) ;
#8353=ORIENTED_EDGE ( 'NONE', *, *, #9166, .F. ) ;
#8357=DIRECTION ( 'NONE',  ( 0.000000000000000000, 0.000000000000000000, 1.000000000000000000 ) ) ;
#8373=EDGE_CURVE ( 'NONE', #763, #10477, #6326, .T. ) ;
#8395=EDGE_CURVE ( 'NONE', #13503, #10710, #452, .T. ) ;
#8416=ORIENTED_EDGE ( 'NONE', *, *, #8395, .T. ) ;
#8418=ORIENTED_EDGE ( 'NONE', *, *, #18190, .T. ) ;
#8425=FACE_OUTER_BOUND ( 'NONE', #15230, .T. ) ;
#8446=ORIENTED_EDGE ( 'NONE', *, *, #8504, .T. ) ;
#8453=AXIS2_PLACEMENT_3D ( 'NONE', #6651, #9850, #15846 ) ;
#8493=VECTOR ( 'NONE', #13105, 1000.000000000000000 ) ;
#8504=EDGE_CURVE ( 'NONE', #6374, #10710, #6438, .T. ) ;
#8511=ADVANCED_FACE ( 'NONE', ( #11025 ), #17027, .T. ) ;
#8516=LINE ( 'NONE', #7138, #8493 ) ;
#8517=CARTESIAN_POINT ( 'NONE',  ( -12.70357423236093197, -43.78611686177728046, 3.000000000000000000 ) ) ;
#8521=FACE_OUTER_BOUND ( 'NONE', #8341, .T. ) ;
#8540=EDGE_LOOP ( 'NONE', ( #5172, #13853, #2332, #9108 ) ) ;
#8558=ORIENTED_EDGE ( 'NONE', *, *, #15200, .F. ) ;
#8561=CARTESIAN_POINT ( 'NONE',  ( -8.528048594804062077, -45.28611686177728046, 3.000000000000000000 ) ) ;
#8629=VERTEX_POINT ( 'NONE', #16186 ) ;
#8654=CARTESIAN_POINT ( 'NONE',  ( -6.528048594804060301, -45.28611686177728046, 1.500000000000000000 ) ) ;
#8665=LINE ( 'NONE', #7395, #9580 ) ;
#8676=EDGE_CURVE ( 'NONE', #8045, #15565, #5159, .T. ) ;
#8680=DIRECTION ( 'NONE',  ( 0.000000000000000000, -0.6139406135149195753, 0.7893522173763268812 ) ) ;
#8684=ORIENTED_EDGE ( 'NONE', *, *, #6199, .F. ) ;
#8688=ORIENTED_EDGE ( 'NONE', *, *, #988, .T. ) ;
#8698=EDGE_LOOP ( 'NONE', ( #12013, #3994, #10460, #14002 ) ) ;
#8711=VECTOR ( 'NONE', #8006, 1000.000000000000000 ) ;
#8751=CARTESIAN_POINT ( 'NONE',  ( -3.155775640247338920, -38.39960408384397539, 3.000000000000000000 ) ) ;
#8774=CARTESIAN_POINT ( 'NONE',  ( -10.00000000000000000, 0.000000000000000000, 1.500000000000000444 ) ) ;
#8775=CARTESIAN_POINT ( 'NONE',  ( 0.000000000000000000, -32.00000000000000711, 1.500000000000000000 ) ) ;
#8800=ORIENTED_EDGE ( 'NONE', *, *, #8676, .F. ) ;
#8805=CARTESIAN_POINT ( 'NONE',  ( -10.00000000000000000, 0.000000000000000000, 7.499999999999995559 ) ) ;
#8807=DIRECTION ( 'NONE',  ( 0.000000000000000000, 1.000000000000000000, 0.000000000000000000 ) ) ;
#8831=DIRECTION ( 'NONE',  ( -0.000000000000000000, -0.000000000000000000, -1.000000000000000000 ) ) ;
#8834=CARTESIAN_POINT ( 'NONE',  ( -15.00000000000000000, 0.000000000000000000, 0.000000000000000000 ) ) ;
#8839=AXIS2_PLACEMENT_3D ( 'NONE', #4403, #10365, #16358 ) ;
#8874=LINE ( 'NONE', #17605, #6561 ) ;
#8908=ORIENTED_EDGE ( 'NONE', *, *, #18567, .T. ) ;
#8913=VECTOR ( 'NONE', #7288, 1000.000000000000000 ) ;
#8916=CARTESIAN_POINT ( 'NONE',  ( 5.421010862427523748E-15, -25.00000000000000711, 0.000000000000000000 ) ) ;
#8938=VECTOR ( 'NONE', #456, 1000.000000000000000 ) ;
#8969=LINE ( 'NONE', #14956, #12972 ) ;
#8979=CARTESIAN_POINT ( 'NONE',  ( -3.065533689247737392, -45.28611686177728046, 3.000000000000000000 ) ) ;
#8992=ORIENTED_EDGE ( 'NONE', *, *, #2352, .T. ) ;
#9001=EDGE_CURVE ( 'NONE', #12626, #16767, #11272, .T. ) ;
#9005=FACE_OUTER_BOUND ( 'NONE', #8019, .T. ) ;
#9025=FACE_OUTER_BOUND ( 'NONE', #13534, .T. ) ;
#9033=CARTESIAN_POINT ( 'NONE',  ( -17.70357423236093553, -43.78611686177728046, 3.000000000000000000 ) ) ;
#9054=CARTESIAN_POINT ( 'NONE',  ( 11.83926609531033058, -43.78611686177728046, 3.000000000000000000 ) ) ;
#9058=AXIS2_PLACEMENT_3D ( 'NONE', #7936, #754, #567 ) ;
#9076=AXIS2_PLACEMENT_3D ( 'NONE', #8240, #16868, #1868 ) ;
#9098=VERTEX_POINT ( 'NONE', #10984 ) ;
#9108=ORIENTED_EDGE ( 'NONE', *, *, #7466, .T. ) ;
#9126=ORIENTED_EDGE ( 'NONE', *, *, #18946, .T. ) ;
#9128=LINE ( 'NONE', #16281, #3919 ) ;
#9136=FACE_OUTER_BOUND ( 'NONE', #19186, .T. ) ;
#9150=LINE ( 'NONE', #1802, #2639 ) ;
#9159=VERTEX_POINT ( 'NONE', #4012 ) ;
#9166=EDGE_CURVE ( 'NONE', #6401, #9696, #17348, .T. ) ;
#9177=DIRECTION ( 'NONE',  ( 0.000000000000000000, 1.000000000000000000, -0.000000000000000000 ) ) ;
#9179=CARTESIAN_POINT ( 'NONE',  ( 11.83926609531033058, -43.78611686177728046, 1.500000000000000000 ) ) ;
#9193=ADVANCED_FACE ( 'NONE', ( #8521 ), #14311, .T. ) ;
#9194=ORIENTED_EDGE ( 'NONE', *, *, #14818, .F. ) ;
#9204=VERTEX_POINT ( 'NONE', #2733 ) ;
#9211=VECTOR ( 'NONE', #3278, 1000.000000000000000 ) ;
#9252=VECTOR ( 'NONE', #14783, 1000.000000000000000 ) ;
#9258=ADVANCED_FACE ( 'NONE', ( #8425 ), #14598, .F. ) ;
#9278=EDGE_CURVE ( 'NONE', #17318, #9490, #6855, .T. ) ;
#9315=ORIENTED_EDGE ( 'NONE', *, *, #17103, .T. ) ;
#9324=DIRECTION ( 'NONE',  ( -0.000000000000000000, 0.000000000000000000, -1.000000000000000000 ) ) ;
#9337=CARTESIAN_POINT ( 'NONE',  ( -3.065533689247737392, -43.60761626555502346, 1.500000000000000000 ) ) ;
#9365=EDGE_LOOP ( 'NONE', ( #14422, #17654, #6676, #11740 ) ) ;
#9389=VECTOR ( 'NONE', #9606, 1000.000000000000000 ) ;
#9390=CARTESIAN_POINT ( 'NONE',  ( -7.999999999999996447, -32.00000000000000711, 0.000000000000000000 ) ) ;
#9393=ORIENTED_EDGE ( 'NONE', *, *, #10563, .T. ) ;
#9409=FACE_OUTER_BOUND ( 'NONE', #8698, .T. ) ;
#9416=CARTESIAN_POINT ( 'NONE',  ( -8.528048594804062077, -42.28611686177728046, 3.000000000000000000 ) ) ;
#9422=CARTESIAN_POINT ( 'NONE',  ( -15.20357423236093375, -43.78611686177728046, 1.500000000000000000 ) ) ;
#9425=CARTESIAN_POINT ( 'NONE',  ( 8.000000000000003553, 0.000000000000000000, 1.500000000000000000 ) ) ;
#9429=LINE ( 'NONE', #17083, #13653 ) ;
#9470=ORIENTED_EDGE ( 'NONE', *, *, #5920, .T. ) ;
#9473=ORIENTED_EDGE ( 'NONE', *, *, #17059, .F. ) ;
#9475=LINE ( 'NONE', #15652, #10501 ) ;
#9480=ORIENTED_EDGE ( 'NONE', *, *, #19218, .T. ) ;
#9489=LINE ( 'NONE', #3331, #17697 ) ;
#9490=VERTEX_POINT ( 'NONE', #10662 ) ;
#9506=VERTEX_POINT ( 'NONE', #2829 ) ;
#9507=CARTESIAN_POINT ( 'NONE',  ( -0.000000000000000000, -52.00000000000000711, 0.000000000000000000 ) ) ;
#9510=FACE_BOUND ( 'NONE', #2157, .T. ) ;
#9517=DIRECTION ( 'NONE',  ( 0.000000000000000000, -0.000000000000000000, -1.000000000000000000 ) ) ;
#9530=ORIENTED_EDGE ( 'NONE', *, *, #11765, .T. ) ;
#9541=VERTEX_POINT ( 'NONE', #13900 ) ;
#9556=AXIS2_PLACEMENT_3D ( 'NONE', #9425, #3257, #9324 ) ;
#9557=DIRECTION ( 'NONE',  ( 0.000000000000000000, 0.000000000000000000, 1.000000000000000000 ) ) ;
#9565=PLANE ( 'NONE',  #6749 ) ;
#9580=VECTOR ( 'NONE', #2689, 1000.000000000000000 ) ;
#9583=VERTEX_POINT ( 'NONE', #8126 ) ;
#9606=DIRECTION ( 'NONE',  ( -0.000000000000000000, -1.000000000000000000, -0.000000000000000000 ) ) ;
#9627=LINE ( 'NONE', #6877, #13768 ) ;
#9629=CARTESIAN_POINT ( 'NONE',  ( -3.155775640247338920, -41.39960408384398249, 3.000000000000000000 ) ) ;
#9636=LINE ( 'NONE', #12673, #18372 ) ;
#9696=VERTEX_POINT ( 'NONE', #9390 ) ;
#9707=ORIENTED_EDGE ( 'NONE', *, *, #2758, .F. ) ;
#9712=CIRCLE ( 'NONE', #8453, 2.500000000000002220 ) ;
#9719=CIRCLE ( 'NONE', #15352, 1.678500596222258556 ) ;
#9727=CARTESIAN_POINT ( 'NONE',  ( -12.50000000000000000, -35.50000000000000000, 1.500000000000000000 ) ) ;
#9730=CYLINDRICAL_SURFACE ( 'NONE', #18384, 2.500000000000002220 ) ;
#9764=PLANE ( 'NONE',  #17848 ) ;
#9770=CARTESIAN_POINT ( 'NONE',  ( -1.485306817036799787, -32.50000000000000711, 1.500000000000000444 ) ) ;
#9783=LINE ( 'NONE', #12912, #13136 ) ;
#9786=EDGE_LOOP ( 'NONE', ( #6874, #4745, #13720, #9393, #10975, #1488, #3833, #14405 ) ) ;
#9792=DIRECTION ( 'NONE',  ( 0.000000000000000000, -1.000000000000000000, 0.000000000000000000 ) ) ;
#9808=ORIENTED_EDGE ( 'NONE', *, *, #1110, .F. ) ;
#9825=VECTOR ( 'NONE', #18943, 1000.000000000000000 ) ;
#9826=CARTESIAN_POINT ( 'NONE',  ( -8.528048594804062077, -45.28611686177728046, 1.500000000000000000 ) ) ;
#9838=EDGE_CURVE ( 'NONE', #8266, #13522, #17885, .T. ) ;
#9850=DIRECTION ( 'NONE',  ( 0.000000000000000000, 0.000000000000000000, 1.000000000000000000 ) ) ;
#9858=EDGE_CURVE ( 'NONE', #9098, #8045, #16044, .T. ) ;
#9874=CARTESIAN_POINT ( 'NONE',  ( -6.528048594804060301, -45.28611686177728046, 3.000000000000000000 ) ) ;
#9899=ORIENTED_EDGE ( 'NONE', *, *, #6546, .F. ) ;
#9902=ORIENTED_EDGE ( 'NONE', *, *, #6772, .T. ) ;
#9910=PRESENTATION_STYLE_ASSIGNMENT (( #5423 ) ) ;
#9926=DIRECTION ( 'NONE',  ( -0.000000000000000000, -0.000000000000000000, -1.000000000000000000 ) ) ;
#9928=EDGE_CURVE ( 'NONE', #16082, #18276, #70, .T. ) ;
#9930=ORIENTED_EDGE ( 'NONE', *, *, #18539, .T. ) ;
#9931=EDGE_CURVE ( 'NONE', #6170, #9506, #15162, .T. ) ;
#9953=VERTEX_POINT ( 'NONE', #2997 ) ;
#9957=AXIS2_PLACEMENT_3D ( 'NONE', #8751, #11788, #1614 ) ;
#9965=ADVANCED_FACE ( 'NONE', ( #5750 ), #10438, .F. ) ;
#9984=EDGE_CURVE ( 'NONE', #18276, #11674, #5850, .T. ) ;
#9996=SHAPE_REPRESENTATION ( 'pcba', ( #1791 ), #3902 ) ;
#10001=AXIS2_PLACEMENT_3D ( 'NONE', #8301, #5550, #18610 ) ;
#10002=DIRECTION ( 'NONE',  ( -0.000000000000000000, -0.000000000000000000, -1.000000000000000000 ) ) ;
#10016=LINE ( 'NONE', #15820, #12515 ) ;
#10050=ORIENTED_EDGE ( 'NONE', *, *, #7396, .F. ) ;
#10075=DIRECTION ( 'NONE',  ( -1.000000000000000000, 0.000000000000000000, 0.000000000000000000 ) ) ;
#10078=VERTEX_POINT ( 'NONE', #15331 ) ;
#10092=CARTESIAN_POINT ( 'NONE',  ( -3.155775640247338920, -41.39960408384398249, 1.500000000000000000 ) ) ;
#10108=LINE ( 'NONE', #12956, #2505 ) ;
#10110=LINE ( 'NONE', #9826, #1881 ) ;
#10135=CARTESIAN_POINT ( 'NONE',  ( -3.155775640247338920, -38.39960408384397539, 1.500000000000000000 ) ) ;
#10136=CARTESIAN_POINT ( 'NONE',  ( -11.75000000000000000, -35.50000000000000000, 5.500000000000000000 ) ) ;
#10154=ORIENTED_EDGE ( 'NONE', *, *, #10715, .F. ) ;
#10187=PRODUCT ( 'pcba', 'pcba', '', ( #10290 ) ) ;
#10198=MANIFOLD_SOLID_BREP ( 'Chamfer1', #14175 ) ;
#10226=LINE ( 'NONE', #2589, #4589 ) ;
#10240=LINE ( 'NONE', #16133, #13422 ) ;
#10247=ORIENTED_EDGE ( 'NONE', *, *, #2934, .T. ) ;
#10281=CIRCLE ( 'NONE', #3726, 1.249999999999999334 ) ;
#10290=PRODUCT_CONTEXT ( 'NONE', #5698, 'mechanical' ) ;
#10329=EDGE_CURVE ( 'NONE', #8266, #763, #18641, .T. ) ;
#10341=DIRECTION ( 'NONE',  ( 1.000000000000000000, 0.000000000000000000, 0.000000000000000000 ) ) ;
#10356=DIRECTION ( 'NONE',  ( 0.000000000000000000, 0.000000000000000000, -1.000000000000000000 ) ) ;
#10358=VECTOR ( 'NONE', #15720, 1000.000000000000000 ) ;
#10365=DIRECTION ( 'NONE',  ( 0.000000000000000000, 0.000000000000000000, -1.000000000000000000 ) ) ;
#10405=LINE ( 'NONE', #1403, #1900 ) ;
#10430=EDGE_CURVE ( 'NONE', #3236, #9583, #5293, .T. ) ;
#10438=PLANE ( 'NONE',  #6912 ) ;
#10448=VERTEX_POINT ( 'NONE', #18729 ) ;
#10449=EDGE_CURVE ( 'NONE', #5590, #10078, #17268, .T. ) ;
#10457=STYLED_ITEM ( 'NONE', ( #7818 ), #4072 ) ;
#10460=ORIENTED_EDGE ( 'NONE', *, *, #13110, .T. ) ;
#10465=EDGE_CURVE ( 'NONE', #8045, #9490, #6949, .T. ) ;
#10477=VERTEX_POINT ( 'NONE', #17343 ) ;
#10501=VECTOR ( 'NONE', #11217, 1000.000000000000000 ) ;
#10518=CARTESIAN_POINT ( 'NONE',  ( -10.00000000000000000, -32.00000000000001421, 3.500000000000006661 ) ) ;
#10526=CIRCLE ( 'NONE', #17111, 2.500000000000000444 ) ;
#10537=LINE ( 'NONE', #8775, #3491 ) ;
#10547=SURFACE_SIDE_STYLE ('',( #8017 ) ) ;
#10563=EDGE_CURVE ( 'NONE', #18251, #301, #8516, .T. ) ;
#10578=FACE_OUTER_BOUND ( 'NONE', #2024, .T. ) ;
#10611=DIRECTION ( 'NONE',  ( -1.000000000000000000, 0.000000000000000000, 0.000000000000000000 ) ) ;
#10638=DIRECTION ( 'NONE',  ( 1.000000000000000000, 0.000000000000000000, 0.000000000000000000 ) ) ;
#10655=ORIENTED_EDGE ( 'NONE', *, *, #8676, .T. ) ;
#10662=CARTESIAN_POINT ( 'NONE',  ( 8.000000000000003553, -32.00000000000000711, 1.500000000000000000 ) ) ;
#10690=AXIS2_PLACEMENT_3D ( 'NONE', #4785, #3584, #9557 ) ;
#10708=ORIENTED_EDGE ( 'NONE', *, *, #1569, .T. ) ;
#10710=VERTEX_POINT ( 'NONE', #16251 ) ;
#10715=EDGE_CURVE ( 'NONE', #4614, #6374, #4869, .T. ) ;
#10742=FILL_AREA_STYLE ('',( #12414 ) ) ;
#10746=CARTESIAN_POINT ( 'NONE',  ( -11.25000000000000178, -35.50000000000000000, 5.500000000000000000 ) ) ;
#10751=EDGE_LOOP ( 'NONE', ( #9902, #5075, #10050, #14208 ) ) ;
#10811=PLANE ( 'NONE',  #12087 ) ;
#10814=UNCERTAINTY_MEASURE_WITH_UNIT (LENGTH_MEASURE( 1.000000000000000082E-05 ), #17192, 'distance_accuracy_value', 'NONE');
#10833=CARTESIAN_POINT ( 'NONE',  ( -6.528048594804060301, -45.28611686177728046, 3.000000000000000000 ) ) ;
#10899=DIRECTION ( 'NONE',  ( 0.000000000000000000, 0.000000000000000000, 1.000000000000000000 ) ) ;
#10902=ORIENTED_EDGE ( 'NONE', *, *, #4853, .F. ) ;
#10952=DIRECTION ( 'NONE',  ( 1.000000000000000000, 0.000000000000000000, 0.000000000000000000 ) ) ;
#10961=ORIENTED_EDGE ( 'NONE', *, *, #5966, .F. ) ;
#10975=ORIENTED_EDGE ( 'NONE', *, *, #7416, .F. ) ;
#10984=CARTESIAN_POINT ( 'NONE',  ( -7.999999999999996447, -25.00000000000000711, 1.500000000000000000 ) ) ;
#10985=VECTOR ( 'NONE', #10952, 1000.000000000000000 ) ;
#10987=PLANE ( 'NONE',  #9556 ) ;
#10997=DIRECTION ( 'NONE',  ( 0.000000000000000000, -0.6139406135149196864, 0.7893522173763268812 ) ) ;
#11013=VECTOR ( 'NONE', #4100, 1000.000000000000000 ) ;
#11025=FACE_OUTER_BOUND ( 'NONE', #11348, .T. ) ;
#11044=VERTEX_POINT ( 'NONE', #5283 ) ;
#11075=DIRECTION ( 'NONE',  ( 0.000000000000000000, -1.000000000000000000, 0.000000000000000000 ) ) ;
#11082=PLANE ( 'NONE',  #1430 ) ;
#11087=AXIS2_PLACEMENT_3D ( 'NONE', #9054, #3074, #10611 ) ;
#11096=DIRECTION ( 'NONE',  ( -1.000000000000000000, 0.000000000000000000, 0.000000000000000000 ) ) ;
#11106=PRODUCT_DEFINITION_FORMATION_WITH_SPECIFIED_SOURCE ( 'ANY', '', #10187, .NOT_KNOWN. ) ;
#11135=VERTEX_POINT ( 'NONE', #18173 ) ;
#11145=CARTESIAN_POINT ( 'NONE',  ( 9.339266095310328808, -43.78611686177728046, 3.000000000000000000 ) ) ;
#11184=EDGE_LOOP ( 'NONE', ( #16373, #7918, #11440, #16464 ) ) ;
#11189=LINE ( 'NONE', #6415, #5666 ) ;
#11193=CARTESIAN_POINT ( 'NONE',  ( -3.065533689247737392, -43.60761626555502346, 3.000000000000000000 ) ) ;
#11217=DIRECTION ( 'NONE',  ( -0.000000000000000000, -0.000000000000000000, -1.000000000000000000 ) ) ;
#11228=EDGE_CURVE ( 'NONE', #9159, #13243, #961, .T. ) ;
#11253=FACE_OUTER_BOUND ( 'NONE', #18015, .T. ) ;
#11265=EDGE_CURVE ( 'NONE', #17053, #11044, #13098, .T. ) ;
#11269=ORIENTED_EDGE ( 'NONE', *, *, #17781, .F. ) ;
#11272=CIRCLE ( 'NONE', #2511, 2.500000000000002220 ) ;
#11283=VECTOR ( 'NONE', #2650, 1000.000000000000000 ) ;
#11289=LINE ( 'NONE', #12946, #9825 ) ;
#11291=FACE_OUTER_BOUND ( 'NONE', #6053, .T. ) ;
#11299=MECHANICAL_DESIGN_GEOMETRIC_PRESENTATION_REPRESENTATION('',(#15086),#3498);
#11303=CARTESIAN_POINT ( 'NONE',  ( -15.00000000000000000, -32.50000000000001421, 3.328446124929187455 ) ) ;
#11315=CARTESIAN_POINT ( 'NONE',  ( 1.753982408753060218, -46.96461745799954457, 3.000000000000000000 ) ) ;
#11317=ORIENTED_EDGE ( 'NONE', *, *, #18832, .T. ) ;
#11348=EDGE_LOOP ( 'NONE', ( #11755, #3336, #12243, #15168 ) ) ;
#11351=CARTESIAN_POINT ( 'NONE',  ( 8.000000000000003553, 0.000000000000000000, 1.500000000000000000 ) ) ;
#11352=CARTESIAN_POINT ( 'NONE',  ( -3.155775640247338920, -41.39960408384398249, 1.500000000000000000 ) ) ;
#11358=EDGE_LOOP ( 'NONE', ( #6577, #3898, #11898, #16478 ) ) ;
#11365=ORIENTED_EDGE ( 'NONE', *, *, #14519, .T. ) ;
#11378=DIRECTION ( 'NONE',  ( 1.000000000000000000, 0.000000000000000000, 0.000000000000000000 ) ) ;
#11401=VECTOR ( 'NONE', #17205, 1000.000000000000000 ) ;
#11427=AXIS2_PLACEMENT_3D ( 'NONE', #7249, #14693, #10075 ) ;
#11440=ORIENTED_EDGE ( 'NONE', *, *, #12384, .T. ) ;
#11446=CIRCLE ( 'NONE', #192, 2.500000000000000444 ) ;
#11451=DIRECTION ( 'NONE',  ( -1.000000000000000000, 0.000000000000000000, 0.000000000000000000 ) ) ;
#11478=ORIENTED_EDGE ( 'NONE', *, *, #13475, .F. ) ;
#11485=ORIENTED_EDGE ( 'NONE', *, *, #7988, .F. ) ;
#11519=CIRCLE ( 'NONE', #10001, 2.500000000000002220 ) ;
#11534=DIRECTION ( 'NONE',  ( 1.000000000000000000, 0.000000000000000000, 0.000000000000000000 ) ) ;
#11546=EDGE_LOOP ( 'NONE', ( #12047, #8688, #18214, #15335 ) ) ;
#11574=CARTESIAN_POINT ( 'NONE',  ( -15.20357423236093375, -43.78611686177728046, 3.000000000000000000 ) ) ;
#11575=EDGE_LOOP ( 'NONE', ( #17172, #5410, #5117, #14808 ) ) ;
#11588=VECTOR ( 'NONE', #4116, 1000.000000000000000 ) ;
#11594=CARTESIAN_POINT ( 'NONE',  ( -3.065533689247737392, -46.96461745799954457, 3.000000000000000000 ) ) ;
#11621=VERTEX_POINT ( 'NONE', #8094 ) ;
#11626=ORIENTED_EDGE ( 'NONE', *, *, #10329, .T. ) ;
#11631=DIRECTION ( 'NONE',  ( -0.000000000000000000, -0.000000000000000000, -1.000000000000000000 ) ) ;
#11634=VERTEX_POINT ( 'NONE', #6625 ) ;
#11644=DIRECTION ( 'NONE',  ( 0.000000000000000000, 0.000000000000000000, -1.000000000000000000 ) ) ;
#11658=ORIENTED_EDGE ( 'NONE', *, *, #5288, .T. ) ;
#11674=VERTEX_POINT ( 'NONE', #15734 ) ;
#11712=CARTESIAN_POINT ( 'NONE',  ( 20.00000000000000355, 0.000000000000000000, 1.500000000000000000 ) ) ;
#11732=DIRECTION ( 'NONE',  ( 0.000000000000000000, -0.6139406135149195753, 0.7893522173763268812 ) ) ;
#11740=ORIENTED_EDGE ( 'NONE', *, *, #2352, .F. ) ;
#11748=EDGE_CURVE ( 'NONE', #11044, #7973, #10110, .T. ) ;
#11749=DIRECTION ( 'NONE',  ( 1.000000000000000000, 2.168404344971008868E-16, 0.000000000000000000 ) ) ;
#11755=ORIENTED_EDGE ( 'NONE', *, *, #9984, .F. ) ;
#11765=EDGE_CURVE ( 'NONE', #14478, #7973, #10016, .T. ) ;
#11771=VECTOR ( 'NONE', #2759, 1000.000000000000000 ) ;
#11784=LINE ( 'NONE', #8654, #6249 ) ;
#11788=DIRECTION ( 'NONE',  ( 0.000000000000000000, -1.000000000000000000, 0.000000000000000000 ) ) ;
#11796=LINE ( 'NONE', #19261, #3330 ) ;
#11816=ORIENTED_EDGE ( 'NONE', *, *, #8201, .T. ) ;
#11822=CARTESIAN_POINT ( 'NONE',  ( -8.528048594804062077, -45.28611686177728046, 3.000000000000000000 ) ) ;
#11855=ORIENTED_EDGE ( 'NONE', *, *, #18746, .F. ) ;
#11864=EDGE_CURVE ( 'NONE', #72, #17032, #16604, .T. ) ;
#11873=AXIS2_PLACEMENT_3D ( 'NONE', #17456, #5415, #3935 ) ;
#11879=ORIENTED_EDGE ( 'NONE', *, *, #11265, .T. ) ;
#11886=CARTESIAN_POINT ( 'NONE',  ( -13.25000000000000178, -35.50000000000000000, 5.500000000000000000 ) ) ;
#11897=VECTOR ( 'NONE', #10997, 1000.000000000000114 ) ;
#11898=ORIENTED_EDGE ( 'NONE', *, *, #16344, .F. ) ;
#11923=EDGE_LOOP ( 'NONE', ( #3554, #9194, #10902, #9530 ) ) ;
#11938=VECTOR ( 'NONE', #6390, 1000.000000000000114 ) ;
#11952=VECTOR ( 'NONE', #18204, 1000.000000000000000 ) ;
#11957=LINE ( 'NONE', #16176, #13437 ) ;
#11965=PLANE ( 'NONE',  #7048 ) ;
#11970=DIRECTION ( 'NONE',  ( 0.000000000000000000, 0.000000000000000000, 1.000000000000000000 ) ) ;
#11978=CARTESIAN_POINT ( 'NONE',  ( -3.065533689247737392, -43.60761626555502346, 1.500000000000000000 ) ) ;
#11984=DIRECTION ( 'NONE',  ( 0.000000000000000000, 1.000000000000000000, -0.000000000000000000 ) ) ;
#12011=CIRCLE ( 'NONE', #14521, 1.249999999999999334 ) ;
#12012=CARTESIAN_POINT ( 'NONE',  ( -19.99999999999999645, -52.00000000000000711, 0.000000000000000000 ) ) ;
#12013=ORIENTED_EDGE ( 'NONE', *, *, #14159, .F. ) ;
#12034=DIRECTION ( 'NONE',  ( 1.000000000000000000, 0.000000000000000000, 0.000000000000000000 ) ) ;
#12047=ORIENTED_EDGE ( 'NONE', *, *, #1569, .F. ) ;
#12052=DIRECTION ( 'NONE',  ( -0.000000000000000000, -0.000000000000000000, -1.000000000000000000 ) ) ;
#12065=CARTESIAN_POINT ( 'NONE',  ( -6.528048594804060301, -45.28611686177728046, 3.000000000000000000 ) ) ;
#12087=AXIS2_PLACEMENT_3D ( 'NONE', #4767, #16713, #3281 ) ;
#12106=DIRECTION ( 'NONE',  ( 0.000000000000000000, 0.000000000000000000, -1.000000000000000000 ) ) ;
#12127=ORIENTED_EDGE ( 'NONE', *, *, #11265, .F. ) ;
#12154=DIRECTION ( 'NONE',  ( -1.000000000000000000, 0.000000000000000000, 0.000000000000000000 ) ) ;
#12155=VERTEX_POINT ( 'NONE', #7781 ) ;
#12160=DIRECTION ( 'NONE',  ( -8.673617379884027583E-16, 1.000000000000000000, 0.000000000000000000 ) ) ;
#12172=AXIS2_PLACEMENT_3D ( 'NONE', #13510, #6070, #12034 ) ;
#12236=CARTESIAN_POINT ( 'NONE',  ( 8.000000000000003553, -25.00000000000000711, 1.500000000000000000 ) ) ;
#12243=ORIENTED_EDGE ( 'NONE', *, *, #13258, .T. ) ;
#12261=ORIENTED_EDGE ( 'NONE', *, *, #19370, .T. ) ;
#12262=CARTESIAN_POINT ( 'NONE',  ( -11.75000000000000000, -35.50000000000000000, 5.500000000000000000 ) ) ;
#12278=ADVANCED_FACE ( 'NONE', ( #6790 ), #5502, .T. ) ;
#12284=DIRECTION ( 'NONE',  ( 1.000000000000000000, 0.000000000000000000, -0.000000000000000000 ) ) ;
#12344=VECTOR ( 'NONE', #10002, 1000.000000000000000 ) ;
#12362=COLOUR_RGB ( '', 0.08235294, 0.09019608, 0.10196078) ;
#12371=UNCERTAINTY_MEASURE_WITH_UNIT (LENGTH_MEASURE( 1.000000000000000082E-05 ), #6446, 'distance_accuracy_value', 'NONE');
#12375=FACE_OUTER_BOUND ( 'NONE', #5757, .T. ) ;
#12384=EDGE_CURVE ( 'NONE', #10477, #15869, #1585, .T. ) ;
#12405=PLANE ( 'NONE',  #14981 ) ;
#12406=CARTESIAN_POINT ( 'NONE',  ( -1.485306817036799787, -37.50000000000000000, 7.499999999999995559 ) ) ;
#12411=ORIENTED_EDGE ( 'NONE', *, *, #17534, .F. ) ;
#12414=FILL_AREA_STYLE_COLOUR ( '', #12362 ) ;
#12431=CARTESIAN_POINT ( 'NONE',  ( -3.065533689247737392, -46.96461745799954457, 3.000000000000000000 ) ) ;
#12448=CARTESIAN_POINT ( 'NONE',  ( 1.753982408753060440, -45.28611686177728046, 1.500000000000000000 ) ) ;
#12458=CARTESIAN_POINT ( 'NONE',  ( -1.485306817036799787, -37.50000000000000000, -3.000000000000000000 ) ) ;
#12459=DIRECTION ( 'NONE',  ( 1.000000000000000000, 0.000000000000000000, -0.000000000000000000 ) ) ;
#12479=CARTESIAN_POINT ( 'NONE',  ( 0.000000000000000000, 0.000000000000000000, 3.000000000000000000 ) ) ;
#12498=PLANE ( 'NONE',  #18439 ) ;
#12515=VECTOR ( 'NONE', #18956, 1000.000000000000000 ) ;
#12519=ORIENTED_EDGE ( 'NONE', *, *, #4697, .T. ) ;
#12575=VECTOR ( 'NONE', #19138, 1000.000000000000000 ) ;
#12580=AXIS2_PLACEMENT_3D ( 'NONE', #15690, #7041, #11534 ) ;
#12595=CARTESIAN_POINT ( 'NONE',  ( -19.99999999999999645, 0.000000000000000000, 1.500000000000000000 ) ) ;
#12600=DIRECTION ( 'NONE',  ( -1.000000000000000000, -8.673617379884027583E-16, 0.000000000000000000 ) ) ;
#12607=ADVANCED_FACE ( 'NONE', ( #9409 ), #16873, .T. ) ;
#12615=FACE_OUTER_BOUND ( 'NONE', #287, .T. ) ;
#12620=EDGE_CURVE ( 'NONE', #13243, #13384, #5954, .T. ) ;
#12623=EDGE_CURVE ( 'NONE', #9541, #9159, #16977, .T. ) ;
#12626=VERTEX_POINT ( 'NONE', #18349 ) ;
#12649=DIRECTION ( 'NONE',  ( 0.000000000000000000, 0.000000000000000000, 1.000000000000000000 ) ) ;
#12665=EDGE_CURVE ( 'NONE', #72, #18276, #3538, .T. ) ;
#12668=( GEOMETRIC_REPRESENTATION_CONTEXT ( 3 ) GLOBAL_UNCERTAINTY_ASSIGNED_CONTEXT ( ( #12371 ) ) GLOBAL_UNIT_ASSIGNED_CONTEXT ( ( #6446, #4881, #13786 ) ) REPRESENTATION_CONTEXT ( 'NONE', 'WORKASPACE' ) );
#12673=CARTESIAN_POINT ( 'NONE',  ( -13.25000000000000178, -35.50000000000000000, 5.500000000000000000 ) ) ;
#12687=CARTESIAN_POINT ( 'NONE',  ( -3.155775640247338920, -41.39960408384398249, 3.000000000000000000 ) ) ;
#12694=CARTESIAN_POINT ( 'NONE',  ( -3.065533689247737392, -45.28611686177728046, 3.000000000000000000 ) ) ;
#12711=VECTOR ( 'NONE', #8072, 1000.000000000000000 ) ;
#12735=CARTESIAN_POINT ( 'NONE',  ( -11.25000000000000178, -35.50000000000000000, 1.500000000000000000 ) ) ;
#12761=( NAMED_UNIT ( * ) SI_UNIT ( $, .STERADIAN. ) SOLID_ANGLE_UNIT ( ) );
#12774=CARTESIAN_POINT ( 'NONE',  ( 1.753982408753060218, -46.96461745799954457, 3.000000000000000000 ) ) ;
#12776=PRODUCT_DEFINITION ( 'UNKNOWN', '', #11106, #13147 ) ;
#12819=ORIENTED_EDGE ( 'NONE', *, *, #10329, .F. ) ;
#12832=LINE ( 'NONE', #15599, #14893 ) ;
#12862=ORIENTED_EDGE ( 'NONE', *, *, #18539, .F. ) ;
#12902=ORIENTED_EDGE ( 'NONE', *, *, #9858, .F. ) ;
#12912=CARTESIAN_POINT ( 'NONE',  ( -3.155775640247338920, -38.39960408384397539, 3.000000000000000000 ) ) ;
#12914=FACE_OUTER_BOUND ( 'NONE', #18153, .T. ) ;
#12926=CARTESIAN_POINT ( 'NONE',  ( -12.50000000000000000, -35.50000000000000000, 5.500000000000000000 ) ) ;
#12946=CARTESIAN_POINT ( 'NONE',  ( -1.485306817036799787, -35.74454190283287147, 7.499999999999995559 ) ) ;
#12956=CARTESIAN_POINT ( 'NONE',  ( 8.000000000000003553, 0.000000000000000000, 0.000000000000000000 ) ) ;
#12972=VECTOR ( 'NONE', #1530, 1000.000000000000000 ) ;
#12979=EDGE_CURVE ( 'NONE', #9696, #15107, #13375, .T. ) ;
#13003=CARTESIAN_POINT ( 'NONE',  ( 1.844224359752661968, -41.39960408384398249, 3.000000000000000000 ) ) ;
#13055=CARTESIAN_POINT ( 'NONE',  ( -0.000000000000000000, -32.00000000000000711, 0.000000000000000000 ) ) ;
#13063=CARTESIAN_POINT ( 'NONE',  ( -3.155775640247338920, -41.39960408384398249, 3.000000000000000000 ) ) ;
#13083=EDGE_CURVE ( 'NONE', #3007, #15605, #18298, .T. ) ;
#13087=ORIENTED_EDGE ( 'NONE', *, *, #8504, .F. ) ;
#13098=LINE ( 'NONE', #19295, #4771 ) ;
#13105=DIRECTION ( 'NONE',  ( 0.000000000000000000, 0.000000000000000000, 1.000000000000000000 ) ) ;
#13110=EDGE_CURVE ( 'NONE', #10448, #3397, #8969, .T. ) ;
#13123=VECTOR ( 'NONE', #11749, 1000.000000000000000 ) ;
#13136=VECTOR ( 'NONE', #18908, 1000.000000000000000 ) ;
#13147=PRODUCT_DEFINITION_CONTEXT ( 'detailed design', #19088, 'design' ) ;
#13159=DIRECTION ( 'NONE',  ( 1.000000000000000000, 0.000000000000000000, 0.000000000000000000 ) ) ;
#13176=ADVANCED_FACE ( 'NONE', ( #3578 ), #6431, .F. ) ;
#13203=ORIENTED_EDGE ( 'NONE', *, *, #10465, .F. ) ;
#13218=EDGE_LOOP ( 'NONE', ( #7022, #8558, #11485, #18619 ) ) ;
#13220=ORIENTED_EDGE ( 'NONE', *, *, #7374, .F. ) ;
#13243=VERTEX_POINT ( 'NONE', #15541 ) ;
#13258=EDGE_CURVE ( 'NONE', #16082, #11634, #14064, .T. ) ;
#13293=CARTESIAN_POINT ( 'NONE',  ( -3.065533689247737392, -46.96461745799954457, 1.500000000000000000 ) ) ;
#13310=ORIENTED_EDGE ( 'NONE', *, *, #18832, .F. ) ;
#13342=EDGE_CURVE ( 'NONE', #17032, #12155, #14637, .T. ) ;
#13350=EDGE_CURVE ( 'NONE', #4393, #4220, #17386, .T. ) ;
#13358=AXIS2_PLACEMENT_3D ( 'NONE', #5983, #15101, #4516 ) ;
#13360=CARTESIAN_POINT ( 'NONE',  ( -15.00000000000000000, 0.000000000000000000, 1.500000000000000444 ) ) ;
#13375=LINE ( 'NONE', #7136, #5631 ) ;
#13379=LINE ( 'NONE', #8774, #5901 ) ;
#13384=VERTEX_POINT ( 'NONE', #7184 ) ;
#13389=ORIENTED_EDGE ( 'NONE', *, *, #2199, .F. ) ;
#13399=FACE_OUTER_BOUND ( 'NONE', #938, .T. ) ;
#13409=ADVANCED_FACE ( 'NONE', ( #17677 ), #16021, .F. ) ;
#13414=ORIENTED_EDGE ( 'NONE', *, *, #10430, .F. ) ;
#13418=DIRECTION ( 'NONE',  ( 0.000000000000000000, -0.6139406135149196864, 0.7893522173763268812 ) ) ;
#13422=VECTOR ( 'NONE', #4480, 1000.000000000000000 ) ;
#13428=DIRECTION ( 'NONE',  ( -2.168404344971008868E-16, 1.000000000000000000, 0.000000000000000000 ) ) ;
#13437=VECTOR ( 'NONE', #2642, 1000.000000000000000 ) ;
#13438=CARTESIAN_POINT ( 'NONE',  ( -3.155775640247338920, -38.39960408384397539, 1.500000000000000000 ) ) ;
#13442=VECTOR ( 'NONE', #2966, 1000.000000000000000 ) ;
#13454=DIRECTION ( 'NONE',  ( 0.000000000000000000, -1.000000000000000000, 0.000000000000000000 ) ) ;
#13466=VERTEX_POINT ( 'NONE', #11303 ) ;
#13475=EDGE_CURVE ( 'NONE', #17318, #17032, #3959, .T. ) ;
#13503=VERTEX_POINT ( 'NONE', #14344 ) ;
#13510=CARTESIAN_POINT ( 'NONE',  ( -3.065533689247737392, -45.28611686177728046, 1.500000000000000000 ) ) ;
#13522=VERTEX_POINT ( 'NONE', #11886 ) ;
#13528=ADVANCED_FACE ( 'NONE', ( #1612 ), #17777, .F. ) ;
#13534=EDGE_LOOP ( 'NONE', ( #1842, #5571, #11658, #8416, #19210, #16072, #1972, #2193 ) ) ;
#13543=DIRECTION ( 'NONE',  ( 0.000000000000000000, 0.000000000000000000, 1.000000000000000000 ) ) ;
#13580=LINE ( 'NONE', #7713, #8938 ) ;
#13597=EDGE_CURVE ( 'NONE', #6401, #9098, #9150, .T. ) ;
#13607=DIRECTION ( 'NONE',  ( -0.000000000000000000, -0.000000000000000000, -1.000000000000000000 ) ) ;
#13611=ORIENTED_EDGE ( 'NONE', *, *, #18567, .F. ) ;
#13653=VECTOR ( 'NONE', #1792, 1000.000000000000000 ) ;
#13658=EDGE_LOOP ( 'NONE', ( #7848, #18378, #13414, #18831 ) ) ;
#13713=CARTESIAN_POINT ( 'NONE',  ( 0.000000000000000000, 0.000000000000000000, 0.000000000000000000 ) ) ;
#13720=ORIENTED_EDGE ( 'NONE', *, *, #18946, .F. ) ;
#13758=FACE_OUTER_BOUND ( 'NONE', #2457, .T. ) ;
#13768=VECTOR ( 'NONE', #8357, 1000.000000000000000 ) ;
#13783=ORIENTED_EDGE ( 'NONE', *, *, #13258, .F. ) ;
#13786=( NAMED_UNIT ( * ) SI_UNIT ( $, .STERADIAN. ) SOLID_ANGLE_UNIT ( ) );
#13798=FACE_OUTER_BOUND ( 'NONE', #16347, .T. ) ;
#13816=ORIENTED_EDGE ( 'NONE', *, *, #13342, .F. ) ;
#13850=PLANE ( 'NONE',  #8170 ) ;
#13853=ORIENTED_EDGE ( 'NONE', *, *, #5654, .F. ) ;
#13883=EDGE_LOOP ( 'NONE', ( #13087, #7582, #14936, #9899 ) ) ;
#13900=CARTESIAN_POINT ( 'NONE',  ( -3.065533689247737392, -46.96461745799954457, 3.000000000000000000 ) ) ;
#13908=ORIENTED_EDGE ( 'NONE', *, *, #13110, .F. ) ;
#13944=LINE ( 'NONE', #519, #11897 ) ;
#13975=DIRECTION ( 'NONE',  ( 1.000000000000000000, 0.000000000000000000, 0.000000000000000000 ) ) ;
#13980=ORIENTED_EDGE ( 'NONE', *, *, #11228, .F. ) ;
#13995=CARTESIAN_POINT ( 'NONE',  ( -15.20357423236093375, -43.78611686177728046, 3.000000000000000000 ) ) ;
#14002=ORIENTED_EDGE ( 'NONE', *, *, #16388, .T. ) ;
#14017=DIRECTION ( 'NONE',  ( 0.000000000000000000, 0.000000000000000000, 1.000000000000000000 ) ) ;
#14020=FACE_BOUND ( 'NONE', #5332, .T. ) ;
#14063=ADVANCED_FACE ( 'NONE', ( #6096 ), #18155, .T. ) ;
#14064=LINE ( 'NONE', #12595, #11401 ) ;
#14072=DIRECTION ( 'NONE',  ( 1.000000000000000000, 0.000000000000000000, 0.000000000000000000 ) ) ;
#14090=ORIENTED_EDGE ( 'NONE', *, *, #6133, .F. ) ;
#14117=VECTOR ( 'NONE', #16530, 1000.000000000000000 ) ;
#14119=ORIENTED_EDGE ( 'NONE', *, *, #15317, .T. ) ;
#14136=ORIENTED_EDGE ( 'NONE', *, *, #4853, .T. ) ;
#14149=LINE ( 'NONE', #15326, #10358 ) ;
#14159=EDGE_CURVE ( 'NONE', #578, #9204, #9128, .T. ) ;
#14160=ADVANCED_FACE ( 'NONE', ( #9025 ), #7458, .T. ) ;
#14174=ADVANCED_FACE ( 'NONE', ( #16386 ), #11965, .T. ) ;
#14175=CLOSED_SHELL ( 'NONE', ( #17577, #17482, #18505, #6544, #16807, #5095, #8511, #9193, #9965, #6998, #17332, #14174, #6598, #7266, #17002, #17149, #12278, #13409, #1060, #2326, #1413, #14547, #2453, #1366, #9258, #17173, #15851, #12607, #16709, #2902, #13528, #3610, #169, #17385, #1851, #14160, #190, #17046, #4081, #16132, #13176, #4607, #14063, #15717, #56 ) ) ;
#14208=ORIENTED_EDGE ( 'NONE', *, *, #16596, .T. ) ;
#14213=ORIENTED_EDGE ( 'NONE', *, *, #12665, .F. ) ;
#14236=CARTESIAN_POINT ( 'NONE',  ( -7.999999999999996447, 0.000000000000000000, 1.500000000000000000 ) ) ;
#14240=CARTESIAN_POINT ( 'NONE',  ( -8.528048594804062077, -42.28611686177728046, 3.000000000000000000 ) ) ;
#14260=FACE_OUTER_BOUND ( 'NONE', #13218, .T. ) ;
#14298=VECTOR ( 'NONE', #199, 1000.000000000000000 ) ;
#14306=DIRECTION ( 'NONE',  ( -0.000000000000000000, -0.000000000000000000, -1.000000000000000000 ) ) ;
#14311=PLANE ( 'NONE',  #15363 ) ;
#14332=PLANE ( 'NONE',  #16809 ) ;
#14333=CARTESIAN_POINT ( 'NONE',  ( 11.83926609531033058, -43.78611686177728046, 3.000000000000000000 ) ) ;
#14344=CARTESIAN_POINT ( 'NONE',  ( -15.00000000000000000, -35.74454190283287147, 7.499999999999995559 ) ) ;
#14376=EDGE_CURVE ( 'NONE', #10477, #763, #3604, .T. ) ;
#14395=DIRECTION ( 'NONE',  ( 0.000000000000000000, 1.000000000000000000, 0.000000000000000000 ) ) ;
#14398=AXIS2_PLACEMENT_3D ( 'NONE', #7760, #7956, #18549 ) ;
#14400=DIRECTION ( 'NONE',  ( 1.000000000000000000, 0.000000000000000000, 0.000000000000000000 ) ) ;
#14405=ORIENTED_EDGE ( 'NONE', *, *, #9166, .T. ) ;
#14422=ORIENTED_EDGE ( 'NONE', *, *, #19218, .F. ) ;
#14427=VECTOR ( 'NONE', #9177, 1000.000000000000000 ) ;
#14432=DIRECTION ( 'NONE',  ( 1.000000000000000000, 0.000000000000000000, 0.000000000000000000 ) ) ;
#14446=CARTESIAN_POINT ( 'NONE',  ( -1.485306817036799787, -35.50000000000000711, 8.000000000000007105 ) ) ;
#14453=DIRECTION ( 'NONE',  ( 0.000000000000000000, 1.000000000000000000, 0.000000000000000000 ) ) ;
#14478=VERTEX_POINT ( 'NONE', #11822 ) ;
#14495=DIRECTION ( 'NONE',  ( -1.000000000000000000, 0.000000000000000000, 0.000000000000000000 ) ) ;
#14519=EDGE_CURVE ( 'NONE', #763, #5273, #4797, .T. ) ;
#14521=AXIS2_PLACEMENT_3D ( 'NONE', #9727, #11970, #6008 ) ;
#14523=DIRECTION ( 'NONE',  ( -0.000000000000000000, 0.000000000000000000, 1.000000000000000000 ) ) ;
#14547=ADVANCED_FACE ( 'NONE', ( #16943 ), #9565, .F. ) ;
#14551=AXIS2_PLACEMENT_3D ( 'NONE', #18117, #10356, #14975 ) ;
#14565=LINE ( 'NONE', #2321, #4335 ) ;
#14593=CARTESIAN_POINT ( 'NONE',  ( -3.155775640247338920, -41.39960408384398249, 3.000000000000000000 ) ) ;
#14597=VECTOR ( 'NONE', #8680, 1000.000000000000227 ) ;
#14598=PLANE ( 'NONE',  #4086 ) ;
#14623=CARTESIAN_POINT ( 'NONE',  ( -8.528048594804062077, -45.28611686177728046, 3.000000000000000000 ) ) ;
#14626=DIRECTION ( 'NONE',  ( -0.000000000000000000, -0.000000000000000000, -1.000000000000000000 ) ) ;
#14627=ORIENTED_EDGE ( 'NONE', *, *, #15356, .F. ) ;
#14636=EDGE_CURVE ( 'NONE', #11634, #11674, #9475, .T. ) ;
#14637=LINE ( 'NONE', #13055, #8913 ) ;
#14693=DIRECTION ( 'NONE',  ( 0.000000000000000000, 0.000000000000000000, -1.000000000000000000 ) ) ;
#14703=AXIS2_PLACEMENT_3D ( 'NONE', #14236, #11096, #2282 ) ;
#14780=ORIENTED_EDGE ( 'NONE', *, *, #5139, .T. ) ;
#14783=DIRECTION ( 'NONE',  ( -0.000000000000000000, -0.000000000000000000, -1.000000000000000000 ) ) ;
#14801=ORIENTED_EDGE ( 'NONE', *, *, #5411, .T. ) ;
#14808=ORIENTED_EDGE ( 'NONE', *, *, #13475, .T. ) ;
#14811=CARTESIAN_POINT ( 'NONE',  ( -10.00000000000000000, -16.78846153846157918, -16.05769230769231015 ) ) ;
#14817=ORIENTED_EDGE ( 'NONE', *, *, #988, .F. ) ;
#14818=EDGE_CURVE ( 'NONE', #3100, #19316, #2734, .T. ) ;
#14822=SHAPE_DEFINITION_REPRESENTATION ( #17890, #9996 ) ;
#14828=ORIENTED_EDGE ( 'NONE', *, *, #3273, .T. ) ;
#14836=ORIENTED_EDGE ( 'NONE', *, *, #17506, .F. ) ;
#14841=PLANE ( 'NONE',  #18811 ) ;
#14893=VECTOR ( 'NONE', #19017, 1000.000000000000000 ) ;
#14901=EDGE_LOOP ( 'NONE', ( #13389, #16693, #492, #10708, #6276, #10154, #4204, #15745 ) ) ;
#14919=CARTESIAN_POINT ( 'NONE',  ( -12.50000000000000000, -35.50000000000000000, 5.500000000000000000 ) ) ;
#14935=CARTESIAN_POINT ( 'NONE',  ( 1.753982408753060440, -43.60761626555502346, 3.000000000000000000 ) ) ;
#14936=ORIENTED_EDGE ( 'NONE', *, *, #9931, .T. ) ;
#14941=CIRCLE ( 'NONE', #13358, 2.500000000000000444 ) ;
#14956=CARTESIAN_POINT ( 'NONE',  ( -3.065533689247737392, -43.60761626555502346, 3.000000000000000000 ) ) ;
#14960=DIRECTION ( 'NONE',  ( 0.000000000000000000, -1.000000000000000000, 0.000000000000000000 ) ) ;
#14964=EDGE_CURVE ( 'NONE', #3236, #17673, #13580, .T. ) ;
#14975=DIRECTION ( 'NONE',  ( 1.000000000000000000, 0.000000000000000000, 0.000000000000000000 ) ) ;
#14981=AXIS2_PLACEMENT_3D ( 'NONE', #10833, #12600, #2118 ) ;
#15007=ORIENTED_EDGE ( 'NONE', *, *, #15732, .F. ) ;
#15025=ORIENTED_EDGE ( 'NONE', *, *, #15732, .T. ) ;
#15065=DIRECTION ( 'NONE',  ( 0.000000000000000000, 0.000000000000000000, 1.000000000000000000 ) ) ;
#15076=EDGE_LOOP ( 'NONE', ( #4120, #3599, #1899, #11855 ) ) ;
#15081=VECTOR ( 'NONE', #6345, 1000.000000000000000 ) ;
#15086=STYLED_ITEM ( 'NONE', ( #9910 ), #10198 ) ;
#15101=DIRECTION ( 'NONE',  ( 0.000000000000000000, 0.000000000000000000, 1.000000000000000000 ) ) ;
#15107=VERTEX_POINT ( 'NONE', #2490 ) ;
#15121=DIRECTION ( 'NONE',  ( 0.000000000000000000, 0.000000000000000000, 1.000000000000000000 ) ) ;
#15162=LINE ( 'NONE', #1538, #4742 ) ;
#15168=ORIENTED_EDGE ( 'NONE', *, *, #14636, .T. ) ;
#15200=EDGE_CURVE ( 'NONE', #856, #13243, #3784, .T. ) ;
#15230=EDGE_LOOP ( 'NONE', ( #2710, #2885, #4294, #11879 ) ) ;
#15256=CARTESIAN_POINT ( 'NONE',  ( -12.50000000000000000, -35.50000000000000000, 5.000000000000003553 ) ) ;
#15289=CARTESIAN_POINT ( 'NONE',  ( 20.00000000000000355, 0.000000000000000000, 1.500000000000000000 ) ) ;
#15317=EDGE_CURVE ( 'NONE', #6543, #17053, #8665, .T. ) ;
#15326=CARTESIAN_POINT ( 'NONE',  ( -1.485306817036799787, -32.00000000000000711, 3.500000000000006661 ) ) ;
#15331=CARTESIAN_POINT ( 'NONE',  ( -12.70357423236093197, -43.78611686177728046, 3.000000000000000000 ) ) ;
#15335=ORIENTED_EDGE ( 'NONE', *, *, #9931, .F. ) ;
#15352=AXIS2_PLACEMENT_3D ( 'NONE', #5620, #15563, #17672 ) ;
#15356=EDGE_CURVE ( 'NONE', #9696, #11674, #10226, .T. ) ;
#15363=AXIS2_PLACEMENT_3D ( 'NONE', #5485, #15880, #7142 ) ;
#15380=FACE_OUTER_BOUND ( 'NONE', #14901, .T. ) ;
#15398=CARTESIAN_POINT ( 'NONE',  ( -10.00000000000000000, -32.00000000000000711, 1.500000000000000000 ) ) ;
#15399=ORIENTED_EDGE ( 'NONE', *, *, #16596, .F. ) ;
#15402=ORIENTED_EDGE ( 'NONE', *, *, #9278, .T. ) ;
#15404=EDGE_CURVE ( 'NONE', #17053, #14478, #11796, .T. ) ;
#15405=CARTESIAN_POINT ( 'NONE',  ( -3.065533689247737392, -46.96461745799954457, 3.000000000000000000 ) ) ;
#15416=DIRECTION ( 'NONE',  ( 1.000000000000000000, 0.000000000000000000, 0.000000000000000000 ) ) ;
#15456=ORIENTED_EDGE ( 'NONE', *, *, #9858, .T. ) ;
#15541=CARTESIAN_POINT ( 'NONE',  ( 1.753982408753060218, -46.96461745799954457, 1.500000000000000000 ) ) ;
#15548=DIRECTION ( 'NONE',  ( 0.000000000000000000, 0.000000000000000000, -1.000000000000000000 ) ) ;
#15563=DIRECTION ( 'NONE',  ( 0.000000000000000000, 0.000000000000000000, 1.000000000000000000 ) ) ;
#15565=VERTEX_POINT ( 'NONE', #1709 ) ;
#15599=CARTESIAN_POINT ( 'NONE',  ( 14.33926609531033058, -43.78611686177728046, 3.000000000000000000 ) ) ;
#15605=VERTEX_POINT ( 'NONE', #10518 ) ;
#15652=CARTESIAN_POINT ( 'NONE',  ( -19.99999999999999645, -32.00000000000000711, 1.500000000000000000 ) ) ;
#15690=CARTESIAN_POINT ( 'NONE',  ( -15.20357423236093375, -43.78611686177728046, 3.000000000000000000 ) ) ;
#15699=LINE ( 'NONE', #2268, #2665 ) ;
#15714=ORIENTED_EDGE ( 'NONE', *, *, #16344, .T. ) ;
#15717=ADVANCED_FACE ( 'NONE', ( #13758 ), #10811, .T. ) ;
#15720=DIRECTION ( 'NONE',  ( -1.000000000000000000, -0.000000000000000000, -0.000000000000000000 ) ) ;
#15732=EDGE_CURVE ( 'NONE', #3523, #10448, #5329, .T. ) ;
#15734=CARTESIAN_POINT ( 'NONE',  ( -19.99999999999999645, -32.00000000000000711, 0.000000000000000000 ) ) ;
#15745=ORIENTED_EDGE ( 'NONE', *, *, #13350, .F. ) ;
#15769=ORIENTED_EDGE ( 'NONE', *, *, #3099, .T. ) ;
#15820=CARTESIAN_POINT ( 'NONE',  ( -8.528048594804062077, -45.28611686177728046, 3.000000000000000000 ) ) ;
#15842=AXIS2_PLACEMENT_3D ( 'NONE', #8979, #7021, #7118 ) ;
#15843=VECTOR ( 'NONE', #2190, 1000.000000000000000 ) ;
#15846=DIRECTION ( 'NONE',  ( 1.000000000000000000, 0.000000000000000000, 0.000000000000000000 ) ) ;
#15851=ADVANCED_FACE ( 'NONE', ( #11291 ), #14332, .F. ) ;
#15869=VERTEX_POINT ( 'NONE', #17372 ) ;
#15880=DIRECTION ( 'NONE',  ( 0.000000000000000000, -1.000000000000000000, 0.000000000000000000 ) ) ;
#15901=FACE_OUTER_BOUND ( 'NONE', #19322, .T. ) ;
#15948=ORIENTED_EDGE ( 'NONE', *, *, #5654, .T. ) ;
#15963=ORIENTED_EDGE ( 'NONE', *, *, #6133, .T. ) ;
#15968=VECTOR ( 'NONE', #13159, 1000.000000000000000 ) ;
#16021=PLANE ( 'NONE',  #17991 ) ;
#16044=LINE ( 'NONE', #2604, #4421 ) ;
#16064=LINE ( 'NONE', #5679, #2472 ) ;
#16070=EDGE_LOOP ( 'NONE', ( #3402, #14780, #12519, #7647 ) ) ;
#16072=ORIENTED_EDGE ( 'NONE', *, *, #1361, .F. ) ;
#16082=VERTEX_POINT ( 'NONE', #3641 ) ;
#16093=CARTESIAN_POINT ( 'NONE',  ( 0.000000000000000000, 0.000000000000000000, 0.000000000000000000 ) ) ;
#16096=DIRECTION ( 'NONE',  ( -1.000000000000000000, 0.000000000000000000, 0.000000000000000000 ) ) ;
#16106=VECTOR ( 'NONE', #17301, 1000.000000000000000 ) ;
#16109=DIRECTION ( 'NONE',  ( -1.000000000000000000, 0.000000000000000000, 0.000000000000000000 ) ) ;
#16132=ADVANCED_FACE ( 'NONE', ( #3731 ), #2267, .T. ) ;
#16133=CARTESIAN_POINT ( 'NONE',  ( 0.000000000000000000, -52.00000000000000711, 1.500000000000000000 ) ) ;
#16148=ORIENTED_EDGE ( 'NONE', *, *, #17534, .T. ) ;
#16172=EDGE_LOOP ( 'NONE', ( #1246, #13908, #15007, #6058 ) ) ;
#16173=ORIENTED_EDGE ( 'NONE', *, *, #11748, .F. ) ;
#16176=CARTESIAN_POINT ( 'NONE',  ( 8.000000000000003553, -32.00000000000000711, 1.500000000000000000 ) ) ;
#16177=ORIENTED_EDGE ( 'NONE', *, *, #4697, .F. ) ;
#16186=CARTESIAN_POINT ( 'NONE',  ( -15.00000000000000000, -35.50000000000000711, 8.000000000000007105 ) ) ;
#16191=FACE_OUTER_BOUND ( 'NONE', #100, .T. ) ;
#16207=LINE ( 'NONE', #13360, #5602 ) ;
#16236=VECTOR ( 'NONE', #11732, 1000.000000000000227 ) ;
#16247=VERTEX_POINT ( 'NONE', #1981 ) ;
#16251=CARTESIAN_POINT ( 'NONE',  ( -15.00000000000000000, -37.50000000000000000, 7.499999999999995559 ) ) ;
#16267=VECTOR ( 'NONE', #12052, 1000.000000000000000 ) ;
#16281=CARTESIAN_POINT ( 'NONE',  ( -4.744034285469996171, -45.28611686177728046, 3.000000000000000000 ) ) ;
#16338=DIRECTION ( 'NONE',  ( -1.000000000000000000, -0.000000000000000000, -0.000000000000000000 ) ) ;
#16344=EDGE_CURVE ( 'NONE', #3100, #6543, #2076, .T. ) ;
#16347=EDGE_LOOP ( 'NONE', ( #5834, #4513, #7657, #4938 ) ) ;
#16348=ORIENTED_EDGE ( 'NONE', *, *, #10430, .T. ) ;
#16358=DIRECTION ( 'NONE',  ( -1.000000000000000000, 0.000000000000000000, 0.000000000000000000 ) ) ;
#16364=EDGE_CURVE ( 'NONE', #301, #8629, #4735, .T. ) ;
#16373=ORIENTED_EDGE ( 'NONE', *, *, #14519, .F. ) ;
#16386=FACE_OUTER_BOUND ( 'NONE', #2630, .T. ) ;
#16388=EDGE_CURVE ( 'NONE', #3397, #9204, #210, .T. ) ;
#16413=DIRECTION ( 'NONE',  ( -1.000000000000000000, 0.000000000000000000, 0.000000000000000000 ) ) ;
#16430=AXIS2_PLACEMENT_3D ( 'NONE', #16706, #6025, #19350 ) ;
#16464=ORIENTED_EDGE ( 'NONE', *, *, #5549, .T. ) ;
#16478=ORIENTED_EDGE ( 'NONE', *, *, #14818, .T. ) ;
#16491=DIRECTION ( 'NONE',  ( 0.000000000000000000, 1.000000000000000000, 0.000000000000000000 ) ) ;
#16494=CARTESIAN_POINT ( 'NONE',  ( 20.00000000000000355, -52.00000000000000711, 1.500000000000000000 ) ) ;
#16530=DIRECTION ( 'NONE',  ( -0.000000000000000000, -0.000000000000000000, -1.000000000000000000 ) ) ;
#16575=CIRCLE ( 'NONE', #12172, 1.678500596222258556 ) ;
#16585=VECTOR ( 'NONE', #9792, 1000.000000000000000 ) ;
#16596=EDGE_CURVE ( 'NONE', #11135, #5165, #5537, .T. ) ;
#16604=LINE ( 'NONE', #5914, #13442 ) ;
#16689=CARTESIAN_POINT ( 'NONE',  ( -15.00000000000000000, -16.78846153846157918, -16.05769230769231015 ) ) ;
#16693=ORIENTED_EDGE ( 'NONE', *, *, #13083, .T. ) ;
#16706=CARTESIAN_POINT ( 'NONE',  ( -3.065533689247737392, -43.60761626555502346, 3.000000000000000000 ) ) ;
#16709=ADVANCED_FACE ( 'NONE', ( #14260 ), #5632, .F. ) ;
#16712=CARTESIAN_POINT ( 'NONE',  ( -8.528048594804062077, -45.28611686177728046, 1.500000000000000000 ) ) ;
#16713=DIRECTION ( 'NONE',  ( 0.000000000000000000, 0.000000000000000000, 1.000000000000000000 ) ) ;
#16735=AXIS2_PLACEMENT_3D ( 'NONE', #16093, #14523, #11378 ) ;
#16767=VERTEX_POINT ( 'NONE', #4558 ) ;
#16807=ADVANCED_FACE ( 'NONE', ( #5925 ), #1707, .T. ) ;
#16809=AXIS2_PLACEMENT_3D ( 'NONE', #12479, #3853, #5424 ) ;
#16822=CARTESIAN_POINT ( 'NONE',  ( -1.485306817036799787, 0.000000000000000000, 7.999999999999996447 ) ) ;
#16868=DIRECTION ( 'NONE',  ( -0.000000000000000000, -0.000000000000000000, -1.000000000000000000 ) ) ;
#16873=CYLINDRICAL_SURFACE ( 'NONE', #14398, 1.678500596222258556 ) ;
#16901=LINE ( 'NONE', #9629, #1294 ) ;
#16920=EDGE_CURVE ( 'NONE', #7973, #19316, #5045, .T. ) ;
#16943=FACE_OUTER_BOUND ( 'NONE', #4957, .T. ) ;
#16977=LINE ( 'NONE', #15405, #2809 ) ;
#16983=CARTESIAN_POINT ( 'NONE',  ( 14.33926609531033058, -43.78611686177728046, 3.000000000000000000 ) ) ;
#17002=ADVANCED_FACE ( 'NONE', ( #18671 ), #17370, .F. ) ;
#17011=DIRECTION ( 'NONE',  ( -0.7071067811865495711, 0.000000000000000000, -0.7071067811865455743 ) ) ;
#17027=PLANE ( 'NONE',  #10690 ) ;
#17032=VERTEX_POINT ( 'NONE', #17285 ) ;
#17046=ADVANCED_FACE ( 'NONE', ( #15901 ), #6701, .T. ) ;
#17053=VERTEX_POINT ( 'NONE', #14240 ) ;
#17054=ORIENTED_EDGE ( 'NONE', *, *, #12620, .T. ) ;
#17059=EDGE_CURVE ( 'NONE', #4614, #13503, #11289, .T. ) ;
#17065=EDGE_CURVE ( 'NONE', #9098, #15107, #18857, .T. ) ;
#17079=AXIS2_PLACEMENT_3D ( 'NONE', #14919, #5897, #3050 ) ;
#17083=CARTESIAN_POINT ( 'NONE',  ( -3.155775640247338920, -41.39960408384398249, 1.500000000000000000 ) ) ;
#17090=VECTOR ( 'NONE', #1269, 1000.000000000000000 ) ;
#17093=DIRECTION ( 'NONE',  ( -0.000000000000000000, -0.000000000000000000, -1.000000000000000000 ) ) ;
#17101=CARTESIAN_POINT ( 'NONE',  ( -10.00000000000000000, -35.50000000000000711, 7.999999999999996447 ) ) ;
#17103=EDGE_CURVE ( 'NONE', #5273, #15869, #12011, .T. ) ;
#17111=AXIS2_PLACEMENT_3D ( 'NONE', #2661, #1008, #14432 ) ;
#17125=AXIS2_PLACEMENT_3D ( 'NONE', #11594, #14453, #1027 ) ;
#17133=CARTESIAN_POINT ( 'NONE',  ( -1.485306817036799787, -16.78846153846157918, -16.05769230769231015 ) ) ;
#17134=CYLINDRICAL_SURFACE ( 'NONE', #4113, 2.500000000000002220 ) ;
#17149=ADVANCED_FACE ( 'NONE', ( #16191 ), #18065, .T. ) ;
#17158=DIRECTION ( 'NONE',  ( 0.000000000000000000, 0.000000000000000000, -1.000000000000000000 ) ) ;
#17172=ORIENTED_EDGE ( 'NONE', *, *, #13342, .T. ) ;
#17173=ADVANCED_FACE ( 'NONE', ( #7570 ), #7368, .F. ) ;
#17188=DIRECTION ( 'NONE',  ( -0.000000000000000000, -0.000000000000000000, -1.000000000000000000 ) ) ;
#17192=( LENGTH_UNIT ( ) NAMED_UNIT ( * ) SI_UNIT ( .MILLI., .METRE. ) );
#17195=VECTOR ( 'NONE', #14306, 1000.000000000000000 ) ;
#17197=ORIENTED_EDGE ( 'NONE', *, *, #5966, .T. ) ;
#17205=DIRECTION ( 'NONE',  ( 0.000000000000000000, 1.000000000000000000, -0.000000000000000000 ) ) ;
#17219=AXIS2_PLACEMENT_3D ( 'NONE', #18668, #17093, #3845 ) ;
#17256=DIRECTION ( 'NONE',  ( -0.000000000000000000, 0.000000000000000000, 1.000000000000000000 ) ) ;
#17268=CIRCLE ( 'NONE', #12580, 2.500000000000002220 ) ;
#17285=CARTESIAN_POINT ( 'NONE',  ( 20.00000000000000355, -32.00000000000000711, 0.000000000000000000 ) ) ;
#17289=ORIENTED_EDGE ( 'NONE', *, *, #8395, .F. ) ;
#17297=CONICAL_SURFACE ( 'NONE', #8839, 0.7500000000000006661, 0.7853981633974511656 ) ;
#17301=DIRECTION ( 'NONE',  ( -0.000000000000000000, -0.000000000000000000, -1.000000000000000000 ) ) ;
#17318=VERTEX_POINT ( 'NONE', #508 ) ;
#17319=DIRECTION ( 'NONE',  ( 0.000000000000000000, -0.7893522173763268812, -0.6139406135149196864 ) ) ;
#17332=ADVANCED_FACE ( 'NONE', ( #9136 ), #10987, .T. ) ;
#17339=PLANE ( 'NONE',  #5362 ) ;
#17343=CARTESIAN_POINT ( 'NONE',  ( -13.75000000000000000, -35.50000000000000000, 5.000000000000003553 ) ) ;
#17348=LINE ( 'NONE', #18918, #11588 ) ;
#17370=PLANE ( 'NONE',  #16735 ) ;
#17372=CARTESIAN_POINT ( 'NONE',  ( -13.75000000000000000, -35.50000000000000000, 1.500000000000000000 ) ) ;
#17385=ADVANCED_FACE ( 'NONE', ( #6594 ), #11082, .T. ) ;
#17386=LINE ( 'NONE', #18871, #19249 ) ;
#17419=DIRECTION ( 'NONE',  ( -1.000000000000000000, -0.000000000000000000, -0.000000000000000000 ) ) ;
#17433=CARTESIAN_POINT ( 'NONE',  ( -9.999999999999996447, -32.50000000000001421, 3.328446124929187455 ) ) ;
#17442=CARTESIAN_POINT ( 'NONE',  ( -8.528048594804062077, -45.28611686177728046, 3.000000000000000000 ) ) ;
#17456=CARTESIAN_POINT ( 'NONE',  ( 11.83926609531033058, -43.78611686177728046, 3.000000000000000000 ) ) ;
#17482=ADVANCED_FACE ( 'NONE', ( #18737 ), #6955, .T. ) ;
#17506=EDGE_CURVE ( 'NONE', #1372, #1647, #12832, .T. ) ;
#17512=VECTOR ( 'NONE', #12154, 1000.000000000000000 ) ;
#17526=EDGE_CURVE ( 'NONE', #6374, #6170, #5303, .T. ) ;
#17534=EDGE_CURVE ( 'NONE', #16247, #11044, #15699, .T. ) ;
#17565=CARTESIAN_POINT ( 'NONE',  ( 8.000000000000003553, -25.00000000000000711, 1.500000000000000000 ) ) ;
#17568=CARTESIAN_POINT ( 'NONE',  ( -1.485306817036799787, -17.18313764714974923, -16.36466261444977377 ) ) ;
#17573=EDGE_LOOP ( 'NONE', ( #12862, #1948 ) ) ;
#17577=ADVANCED_FACE ( 'NONE', ( #9005 ), #4561, .T. ) ;
#17605=CARTESIAN_POINT ( 'NONE',  ( -3.155775640247338920, -38.39960408384397539, 3.000000000000000000 ) ) ;
#17654=ORIENTED_EDGE ( 'NONE', *, *, #17506, .T. ) ;
#17672=DIRECTION ( 'NONE',  ( 1.000000000000000000, 0.000000000000000000, 0.000000000000000000 ) ) ;
#17673=VERTEX_POINT ( 'NONE', #4411 ) ;
#17677=FACE_OUTER_BOUND ( 'NONE', #13658, .T. ) ;
#17697=VECTOR ( 'NONE', #13607, 1000.000000000000000 ) ;
#17733=CARTESIAN_POINT ( 'NONE',  ( 0.000000000000000000, -32.00000000000000711, 1.500000000000000000 ) ) ;
#17777=PLANE ( 'NONE',  #16430 ) ;
#17781=EDGE_CURVE ( 'NONE', #3523, #13384, #9489, .T. ) ;
#17815=ORIENTED_EDGE ( 'NONE', *, *, #5549, .F. ) ;
#17842=LINE ( 'NONE', #15289, #14298 ) ;
#17844=CIRCLE ( 'NONE', #5322, 0.7500000000000006661 ) ;
#17848=AXIS2_PLACEMENT_3D ( 'NONE', #17133, #17319, #2229 ) ;
#17870=ORIENTED_EDGE ( 'NONE', *, *, #9928, .T. ) ;
#17885=CIRCLE ( 'NONE', #18816, 0.7500000000000006661 ) ;
#17890=PRODUCT_DEFINITION_SHAPE ( 'NONE', 'NONE',  #12776 ) ;
#17901=EDGE_CURVE ( 'NONE', #4393, #11621, #5272, .T. ) ;
#17942=ORIENTED_EDGE ( 'NONE', *, *, #14159, .T. ) ;
#17991=AXIS2_PLACEMENT_3D ( 'NONE', #1111, #16109, #2580 ) ;
#17999=DIRECTION ( 'NONE',  ( -0.000000000000000000, 0.000000000000000000, 1.000000000000000000 ) ) ;
#18008=CARTESIAN_POINT ( 'NONE',  ( -19.99999999999999645, 0.000000000000000000, 0.000000000000000000 ) ) ;
#18014=PLANE ( 'NONE',  #7532 ) ;
#18015=EDGE_LOOP ( 'NONE', ( #11816, #2570, #6870, #9808, #9126, #13783, #8264, #12261, #15402, #13203, #12902, #8235 ) ) ;
#18016=EDGE_LOOP ( 'NONE', ( #7477, #11478, #18338, #5993 ) ) ;
#18051=VERTEX_POINT ( 'NONE', #11145 ) ;
#18065=CYLINDRICAL_SURFACE ( 'NONE', #5150, 2.500000000000000444 ) ;
#18070=AXIS2_PLACEMENT_3D ( 'NONE', #19279, #15065, #10341 ) ;
#18117=CARTESIAN_POINT ( 'NONE',  ( -12.50000000000000000, -35.50000000000000000, 5.000000000000003553 ) ) ;
#18146=LINE ( 'NONE', #14811, #18177 ) ;
#18153=EDGE_LOOP ( 'NONE', ( #9473, #2133, #8446, #17289 ) ) ;
#18155=CYLINDRICAL_SURFACE ( 'NONE', #17079, 1.249999999999999334 ) ;
#18173=CARTESIAN_POINT ( 'NONE',  ( -3.155775640247338920, -41.39960408384398249, 3.000000000000000000 ) ) ;
#18176=ORIENTED_EDGE ( 'NONE', *, *, #18394, .F. ) ;
#18177=VECTOR ( 'NONE', #13418, 1000.000000000000114 ) ;
#18190=EDGE_CURVE ( 'NONE', #10448, #578, #6464, .T. ) ;
#18204=DIRECTION ( 'NONE',  ( 0.000000000000000000, -1.000000000000000000, 0.000000000000000000 ) ) ;
#18214=ORIENTED_EDGE ( 'NONE', *, *, #1361, .T. ) ;
#18218=ORIENTED_EDGE ( 'NONE', *, *, #16388, .F. ) ;
#18226=EDGE_LOOP ( 'NONE', ( #14090, #17942, #14801, #5952 ) ) ;
#18229=CARTESIAN_POINT ( 'NONE',  ( -15.00000000000000000, -32.00000000000000711, 3.500000000000006661 ) ) ;
#18237=ORIENTED_EDGE ( 'NONE', *, *, #4960, .T. ) ;
#18251=VERTEX_POINT ( 'NONE', #1239 ) ;
#18276=VERTEX_POINT ( 'NONE', #12012 ) ;
#18298=LINE ( 'NONE', #1821, #6723 ) ;
#18323=MECHANICAL_DESIGN_GEOMETRIC_PRESENTATION_REPRESENTATION('',(#10457),#12668);
#18338=ORIENTED_EDGE ( 'NONE', *, *, #19370, .F. ) ;
#18349=CARTESIAN_POINT ( 'NONE',  ( -17.70357423236093553, -43.78611686177728046, 1.500000000000000000 ) ) ;
#18362=EDGE_CURVE ( 'NONE', #1647, #793, #11446, .T. ) ;
#18372=VECTOR ( 'NONE', #17011, 1000.000000000000114 ) ;
#18378=ORIENTED_EDGE ( 'NONE', *, *, #7466, .F. ) ;
#18379=CARTESIAN_POINT ( 'NONE',  ( -10.00000000000000000, -37.50000000000000000, 7.499999999999995559 ) ) ;
#18384=AXIS2_PLACEMENT_3D ( 'NONE', #11574, #14626, #16096 ) ;
#18388=ORIENTED_EDGE ( 'NONE', *, *, #5288, .F. ) ;
#18394=EDGE_CURVE ( 'NONE', #13522, #10477, #9636, .T. ) ;
#18409=VERTEX_POINT ( 'NONE', #17101 ) ;
#18411=SURFACE_STYLE_USAGE ( .BOTH. , #10547 ) ;
#18439=AXIS2_PLACEMENT_3D ( 'NONE', #12687, #13975, #15548 ) ;
#18445=DIRECTION ( 'NONE',  ( -0.000000000000000000, -0.000000000000000000, -1.000000000000000000 ) ) ;
#18474=LINE ( 'NONE', #9337, #6619 ) ;
#18505=ADVANCED_FACE ( 'NONE', ( #8273 ), #9730, .T. ) ;
#18522=DIRECTION ( 'NONE',  ( -1.000000000000000000, 0.000000000000000000, 0.000000000000000000 ) ) ;
#18539=EDGE_CURVE ( 'NONE', #793, #1647, #10526, .T. ) ;
#18541=COLOUR_RGB ( '', 0.08235294, 0.09019608, 0.10196078) ;
#18549=DIRECTION ( 'NONE',  ( -1.000000000000000000, 0.000000000000000000, 0.000000000000000000 ) ) ;
#18567=EDGE_CURVE ( 'NONE', #18051, #1372, #19304, .T. ) ;
#18588=CARTESIAN_POINT ( 'NONE',  ( 9.339266095310328808, -43.78611686177728046, 1.500000000000000000 ) ) ;
#18610=DIRECTION ( 'NONE',  ( 1.000000000000000000, 0.000000000000000000, 0.000000000000000000 ) ) ;
#18619=ORIENTED_EDGE ( 'NONE', *, *, #12623, .T. ) ;
#18637=EDGE_CURVE ( 'NONE', #5590, #12626, #6105, .T. ) ;
#18641=LINE ( 'NONE', #12262, #11938 ) ;
#18668=CARTESIAN_POINT ( 'NONE',  ( -3.065533689247737392, -45.28611686177728046, 3.000000000000000000 ) ) ;
#18671=FACE_OUTER_BOUND ( 'NONE', #7884, .T. ) ;
#18698=DIRECTION ( 'NONE',  ( 0.000000000000000000, 0.000000000000000000, 1.000000000000000000 ) ) ;
#18704=CARTESIAN_POINT ( 'NONE',  ( 1.844224359752661968, -41.39960408384398249, 1.500000000000000000 ) ) ;
#18722=VERTEX_POINT ( 'NONE', #16494 ) ;
#18726=ORIENTED_EDGE ( 'NONE', *, *, #7988, .T. ) ;
#18729=CARTESIAN_POINT ( 'NONE',  ( -3.065533689247737392, -43.60761626555502346, 3.000000000000000000 ) ) ;
#18737=FACE_OUTER_BOUND ( 'NONE', #893, .T. ) ;
#18744=EDGE_CURVE ( 'NONE', #6113, #2052, #5905, .T. ) ;
#18746=EDGE_CURVE ( 'NONE', #11621, #13466, #7573, .T. ) ;
#18811=AXIS2_PLACEMENT_3D ( 'NONE', #1412, #13454, #4761 ) ;
#18816=AXIS2_PLACEMENT_3D ( 'NONE', #850, #6830, #7117 ) ;
#18830=ORIENTED_EDGE ( 'NONE', *, *, #18744, .F. ) ;
#18831=ORIENTED_EDGE ( 'NONE', *, *, #14964, .T. ) ;
#18832=EDGE_CURVE ( 'NONE', #2052, #5165, #9429, .T. ) ;
#18849=FACE_OUTER_BOUND ( 'NONE', #330, .T. ) ;
#18857=LINE ( 'NONE', #5239, #12344 ) ;
#18871=CARTESIAN_POINT ( 'NONE',  ( -10.00000000000000000, -32.50000000000000711, -3.000000000000000000 ) ) ;
#18885=DIRECTION ( 'NONE',  ( 1.000000000000000000, 0.000000000000000000, 0.000000000000000000 ) ) ;
#18908=DIRECTION ( 'NONE',  ( -1.000000000000000000, -0.000000000000000000, -0.000000000000000000 ) ) ;
#18915=FACE_BOUND ( 'NONE', #17573, .T. ) ;
#18918=CARTESIAN_POINT ( 'NONE',  ( -7.999999999999996447, -32.00000000000000711, 1.500000000000000000 ) ) ;
#18920=DIRECTION ( 'NONE',  ( -0.000000000000000000, -0.000000000000000000, -1.000000000000000000 ) ) ;
#18943=DIRECTION ( 'NONE',  ( -1.000000000000000000, -0.000000000000000000, -0.000000000000000000 ) ) ;
#18946=EDGE_CURVE ( 'NONE', #18251, #11634, #8161, .T. ) ;
#18950=AXIS2_PLACEMENT_3D ( 'NONE', #14623, #16491, #2859 ) ;
#18956=DIRECTION ( 'NONE',  ( -0.000000000000000000, -0.000000000000000000, -1.000000000000000000 ) ) ;
#18982=DIRECTION ( 'NONE',  ( 0.000000000000000000, 1.000000000000000000, 0.000000000000000000 ) ) ;
#18989=VECTOR ( 'NONE', #12160, 1000.000000000000000 ) ;
#18993=ORIENTED_EDGE ( 'NONE', *, *, #15404, .T. ) ;
#19010=ORIENTED_EDGE ( 'NONE', *, *, #4719, .T. ) ;
#19017=DIRECTION ( 'NONE',  ( -0.000000000000000000, -0.000000000000000000, -1.000000000000000000 ) ) ;
#19033=LINE ( 'NONE', #10092, #11283 ) ;
#19041=ORIENTED_EDGE ( 'NONE', *, *, #2934, .F. ) ;
#19088=APPLICATION_CONTEXT ( 'automotive_design' ) ;
#19103=VECTOR ( 'NONE', #18982, 1000.000000000000000 ) ;
#19138=DIRECTION ( 'NONE',  ( -0.000000000000000000, -0.000000000000000000, -1.000000000000000000 ) ) ;
#19174=CARTESIAN_POINT ( 'NONE',  ( -4.744034285469996171, -45.28611686177728046, 3.000000000000000000 ) ) ;
#19186=EDGE_LOOP ( 'NONE', ( #4523, #8800, #1764, #9470 ) ) ;
#19210=ORIENTED_EDGE ( 'NONE', *, *, #6546, .T. ) ;
#19218=EDGE_CURVE ( 'NONE', #1372, #18051, #14941, .T. ) ;
#19249=VECTOR ( 'NONE', #2479, 1000.000000000000000 ) ;
#19255=FACE_OUTER_BOUND ( 'NONE', #8540, .T. ) ;
#19261=CARTESIAN_POINT ( 'NONE',  ( -8.528048594804062077, -45.28611686177728046, 3.000000000000000000 ) ) ;
#19279=CARTESIAN_POINT ( 'NONE',  ( -3.065533689247737392, -45.28611686177728046, 1.500000000000000000 ) ) ;
#19295=CARTESIAN_POINT ( 'NONE',  ( -8.528048594804062077, -42.28611686177728046, 3.000000000000000000 ) ) ;
#19304=CIRCLE ( 'NONE', #3960, 2.500000000000000444 ) ;
#19316=VERTEX_POINT ( 'NONE', #7444 ) ;
#19322=EDGE_LOOP ( 'NONE', ( #6649, #6366, #4213, #18388 ) ) ;
#19350=DIRECTION ( 'NONE',  ( 0.000000000000000000, -0.000000000000000000, -1.000000000000000000 ) ) ;
#19370=EDGE_CURVE ( 'NONE', #18722, #17318, #17842, .T. ) ;
#19383=DIRECTION ( 'NONE',  ( 0.000000000000000000, -0.000000000000000000, -1.000000000000000000 ) ) ;
#19384=ORIENTED_EDGE ( 'NONE', *, *, #16364, .T. ) ;
ENDSEC;
END-ISO-10303-21;
